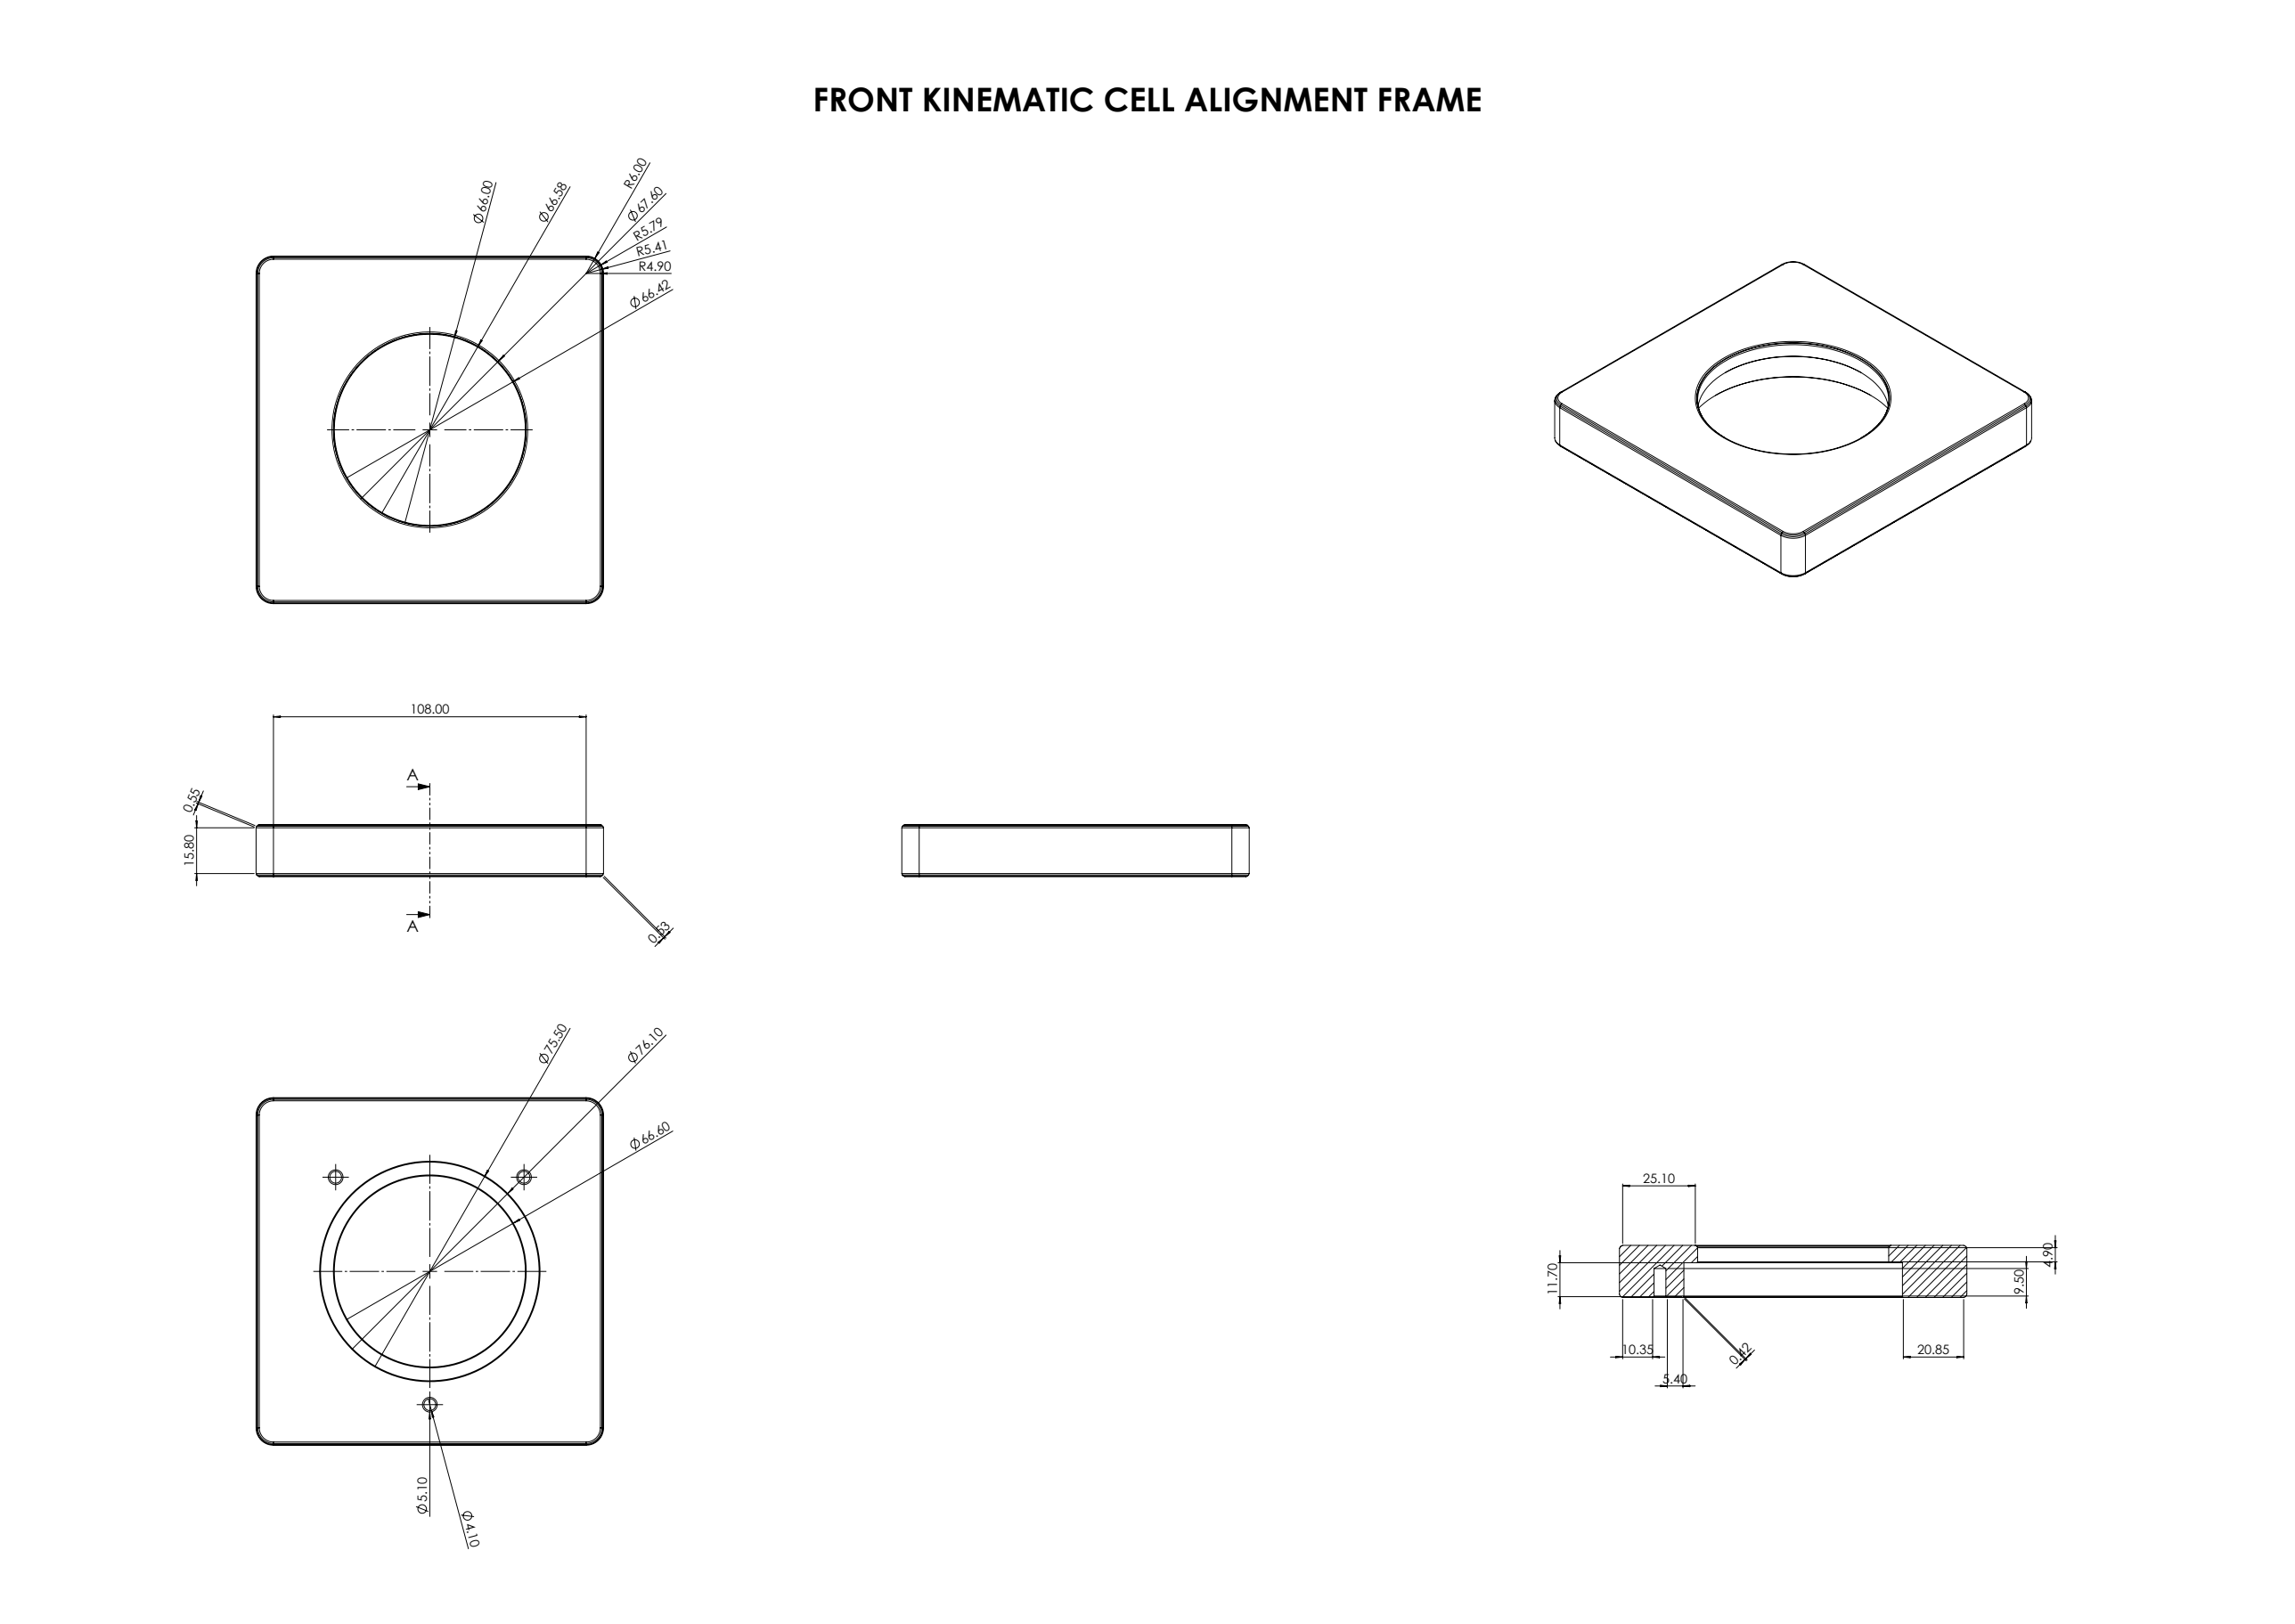
ISO-10303-21;
HEADER;
/* Generated by software containing ST-Developer
 * from STEP Tools, Inc. (www.steptools.com) 
 */

FILE_DESCRIPTION(
/* description */ (''),
/* implementation_level */ '2;1');

FILE_NAME(
/* name */ '03_Front_Kinematic_Cell_Alignment_Frame.step',
/* time_stamp */ '2026-10-19T22:59:19-07:00',
/* author */ (''),
/* organization */ (''),
/* preprocessor_version */ 'ST-DEVELOPER v20.2',
/* originating_system */ 'Autodesk Translation Framework v15.15.0.0',
/* authorisation */ '');

FILE_SCHEMA (('AUTOMOTIVE_DESIGN { 1 0 10303 214 3 1 1 }'));
ENDSEC;

DATA;
#10=MECHANICAL_DESIGN_GEOMETRIC_PRESENTATION_REPRESENTATION('',(#913),#53650);
#881=SHAPE_REPRESENTATION_RELATIONSHIP('SRR','None',#53726,#897);
#897=ADVANCED_BREP_SHAPE_REPRESENTATION('',(#929),#53636);
#913=STYLED_ITEM('',(#53937),#929);
#929=MANIFOLD_SOLID_BREP('Front Cell Alignment Frame',#23305);
#978=CYLINDRICAL_SURFACE('',#23898,0.6);
#979=CYLINDRICAL_SURFACE('',#23901,0.6);
#980=CYLINDRICAL_SURFACE('',#23929,3.775);
#981=CYLINDRICAL_SURFACE('',#23953,3.3);
#982=CYLINDRICAL_SURFACE('',#23963,0.205);
#983=CYLINDRICAL_SURFACE('',#23968,0.205);
#984=CYLINDRICAL_SURFACE('',#23973,0.205);
#985=CYLINDRICAL_SURFACE('',#23980,0.6);
#986=CYLINDRICAL_SURFACE('',#23982,0.6);
#1320=FACE_BOUND('',#3813,.T.);
#1321=FACE_BOUND('',#3814,.T.);
#1322=FACE_BOUND('',#3815,.T.);
#1323=FACE_BOUND('',#3816,.T.);
#1324=FACE_BOUND('',#3857,.T.);
#1325=FACE_BOUND('',#3861,.T.);
#1518=PLANE('',#23860);
#1519=PLANE('',#23864);
#1520=PLANE('',#23868);
#1521=PLANE('',#23872);
#1522=PLANE('',#23873);
#1523=PLANE('',#23876);
#1524=PLANE('',#23879);
#1525=PLANE('',#23884);
#1526=PLANE('',#23888);
#1527=PLANE('',#23891);
#1528=PLANE('',#23894);
#1529=PLANE('',#23900);
#1530=PLANE('',#23903);
#1531=PLANE('',#23905);
#1532=PLANE('',#23908);
#1533=PLANE('',#23911);
#1534=PLANE('',#23915);
#1535=PLANE('',#23919);
#1536=PLANE('',#23920);
#1537=PLANE('',#23923);
#1538=PLANE('',#23933);
#1539=PLANE('',#23936);
#1540=PLANE('',#23940);
#1541=PLANE('',#23944);
#1542=PLANE('',#23945);
#1543=PLANE('',#23947);
#1544=PLANE('',#23948);
#1545=PLANE('',#23955);
#1546=PLANE('',#23977);
#1547=PLANE('',#23979);
#1548=PLANE('',#23981);
#2429=FACE_OUTER_BOUND('',#3800,.T.);
#2430=FACE_OUTER_BOUND('',#3801,.T.);
#2431=FACE_OUTER_BOUND('',#3802,.T.);
#2432=FACE_OUTER_BOUND('',#3803,.T.);
#2433=FACE_OUTER_BOUND('',#3804,.T.);
#2434=FACE_OUTER_BOUND('',#3805,.T.);
#2435=FACE_OUTER_BOUND('',#3806,.T.);
#2436=FACE_OUTER_BOUND('',#3807,.T.);
#2437=FACE_OUTER_BOUND('',#3808,.T.);
#2438=FACE_OUTER_BOUND('',#3809,.T.);
#2439=FACE_OUTER_BOUND('',#3810,.T.);
#2440=FACE_OUTER_BOUND('',#3811,.T.);
#2441=FACE_OUTER_BOUND('',#3812,.T.);
#2442=FACE_OUTER_BOUND('',#3817,.T.);
#2443=FACE_OUTER_BOUND('',#3818,.T.);
#2444=FACE_OUTER_BOUND('',#3819,.T.);
#2445=FACE_OUTER_BOUND('',#3820,.T.);
#2446=FACE_OUTER_BOUND('',#3821,.T.);
#2447=FACE_OUTER_BOUND('',#3822,.T.);
#2448=FACE_OUTER_BOUND('',#3823,.T.);
#2449=FACE_OUTER_BOUND('',#3824,.T.);
#2450=FACE_OUTER_BOUND('',#3825,.T.);
#2451=FACE_OUTER_BOUND('',#3826,.T.);
#2452=FACE_OUTER_BOUND('',#3827,.T.);
#2453=FACE_OUTER_BOUND('',#3828,.T.);
#2454=FACE_OUTER_BOUND('',#3829,.T.);
#2455=FACE_OUTER_BOUND('',#3830,.T.);
#2456=FACE_OUTER_BOUND('',#3831,.T.);
#2457=FACE_OUTER_BOUND('',#3832,.T.);
#2458=FACE_OUTER_BOUND('',#3833,.T.);
#2459=FACE_OUTER_BOUND('',#3834,.T.);
#2460=FACE_OUTER_BOUND('',#3835,.T.);
#2461=FACE_OUTER_BOUND('',#3836,.T.);
#2462=FACE_OUTER_BOUND('',#3837,.T.);
#2463=FACE_OUTER_BOUND('',#3838,.T.);
#2464=FACE_OUTER_BOUND('',#3839,.T.);
#2465=FACE_OUTER_BOUND('',#3840,.T.);
#2466=FACE_OUTER_BOUND('',#3841,.T.);
#2467=FACE_OUTER_BOUND('',#3842,.T.);
#2468=FACE_OUTER_BOUND('',#3843,.T.);
#2469=FACE_OUTER_BOUND('',#3844,.T.);
#2470=FACE_OUTER_BOUND('',#3845,.T.);
#2471=FACE_OUTER_BOUND('',#3846,.T.);
#2472=FACE_OUTER_BOUND('',#3847,.T.);
#2473=FACE_OUTER_BOUND('',#3848,.T.);
#2474=FACE_OUTER_BOUND('',#3849,.T.);
#2475=FACE_OUTER_BOUND('',#3850,.T.);
#2476=FACE_OUTER_BOUND('',#3851,.T.);
#2477=FACE_OUTER_BOUND('',#3852,.T.);
#2478=FACE_OUTER_BOUND('',#3853,.T.);
#2479=FACE_OUTER_BOUND('',#3854,.T.);
#2480=FACE_OUTER_BOUND('',#3855,.T.);
#2481=FACE_OUTER_BOUND('',#3856,.T.);
#2482=FACE_OUTER_BOUND('',#3858,.T.);
#2483=FACE_OUTER_BOUND('',#3859,.T.);
#2484=FACE_OUTER_BOUND('',#3860,.T.);
#2485=FACE_OUTER_BOUND('',#3862,.T.);
#2486=FACE_OUTER_BOUND('',#3863,.T.);
#2487=FACE_OUTER_BOUND('',#3864,.T.);
#2488=FACE_OUTER_BOUND('',#3865,.T.);
#2489=FACE_OUTER_BOUND('',#3866,.T.);
#2490=FACE_OUTER_BOUND('',#3867,.T.);
#2491=FACE_OUTER_BOUND('',#3868,.T.);
#2492=FACE_OUTER_BOUND('',#3869,.T.);
#2493=FACE_OUTER_BOUND('',#3870,.T.);
#2494=FACE_OUTER_BOUND('',#3871,.T.);
#2495=FACE_OUTER_BOUND('',#3872,.T.);
#2496=FACE_OUTER_BOUND('',#3873,.T.);
#2497=FACE_OUTER_BOUND('',#3874,.T.);
#2498=FACE_OUTER_BOUND('',#3875,.T.);
#2499=FACE_OUTER_BOUND('',#3876,.T.);
#2500=FACE_OUTER_BOUND('',#3877,.T.);
#2501=FACE_OUTER_BOUND('',#3878,.T.);
#2502=FACE_OUTER_BOUND('',#3879,.T.);
#2503=FACE_OUTER_BOUND('',#3880,.T.);
#3800=EDGE_LOOP('',(#15901,#15902,#15903,#15904));
#3801=EDGE_LOOP('',(#15905,#15906,#15907,#15908));
#3802=EDGE_LOOP('',(#15909,#15910,#15911,#15912));
#3803=EDGE_LOOP('',(#15913,#15914,#15915,#15916));
#3804=EDGE_LOOP('',(#15917,#15918,#15919,#15920));
#3805=EDGE_LOOP('',(#15921,#15922,#15923,#15924));
#3806=EDGE_LOOP('',(#15925,#15926,#15927,#15928));
#3807=EDGE_LOOP('',(#15929,#15930,#15931,#15932));
#3808=EDGE_LOOP('',(#15933,#15934,#15935,#15936));
#3809=EDGE_LOOP('',(#15937,#15938,#15939,#15940));
#3810=EDGE_LOOP('',(#15941,#15942,#15943,#15944));
#3811=EDGE_LOOP('',(#15945,#15946,#15947,#15948));
#3812=EDGE_LOOP('',(#15949,#15950,#15951,#15952,#15953,#15954,#15955,#15956));
#3813=EDGE_LOOP('',(#15957));
#3814=EDGE_LOOP('',(#15958));
#3815=EDGE_LOOP('',(#15959));
#3816=EDGE_LOOP('',(#15960));
#3817=EDGE_LOOP('',(#15961,#15962,#15963,#15964));
#3818=EDGE_LOOP('',(#15965,#15966,#15967,#15968));
#3819=EDGE_LOOP('',(#15969,#15970,#15971,#15972));
#3820=EDGE_LOOP('',(#15973,#15974,#15975,#15976));
#3821=EDGE_LOOP('',(#15977,#15978,#15979,#15980));
#3822=EDGE_LOOP('',(#15981,#15982,#15983,#15984));
#3823=EDGE_LOOP('',(#15985,#15986,#15987,#15988));
#3824=EDGE_LOOP('',(#15989,#15990,#15991,#15992));
#3825=EDGE_LOOP('',(#15993,#15994,#15995,#15996));
#3826=EDGE_LOOP('',(#15997,#15998,#15999,#16000));
#3827=EDGE_LOOP('',(#16001,#16002,#16003,#16004));
#3828=EDGE_LOOP('',(#16005,#16006,#16007,#16008));
#3829=EDGE_LOOP('',(#16009,#16010,#16011,#16012));
#3830=EDGE_LOOP('',(#16013,#16014,#16015,#16016));
#3831=EDGE_LOOP('',(#16017,#16018,#16019,#16020));
#3832=EDGE_LOOP('',(#16021,#16022,#16023,#16024));
#3833=EDGE_LOOP('',(#16025,#16026,#16027,#16028));
#3834=EDGE_LOOP('',(#16029,#16030,#16031,#16032));
#3835=EDGE_LOOP('',(#16033,#16034,#16035,#16036));
#3836=EDGE_LOOP('',(#16037,#16038,#16039,#16040));
#3837=EDGE_LOOP('',(#16041,#16042,#16043,#16044));
#3838=EDGE_LOOP('',(#16045,#16046,#16047,#16048));
#3839=EDGE_LOOP('',(#16049,#16050,#16051,#16052));
#3840=EDGE_LOOP('',(#16053,#16054,#16055,#16056));
#3841=EDGE_LOOP('',(#16057,#16058,#16059,#16060));
#3842=EDGE_LOOP('',(#16061,#16062,#16063,#16064));
#3843=EDGE_LOOP('',(#16065,#16066,#16067,#16068,#16069));
#3844=EDGE_LOOP('',(#16070,#16071,#16072,#16073,#16074));
#3845=EDGE_LOOP('',(#16075,#16076,#16077,#16078));
#3846=EDGE_LOOP('',(#16079,#16080,#16081,#16082));
#3847=EDGE_LOOP('',(#16083,#16084,#16085,#16086));
#3848=EDGE_LOOP('',(#16087,#16088,#16089,#16090));
#3849=EDGE_LOOP('',(#16091,#16092,#16093,#16094));
#3850=EDGE_LOOP('',(#16095,#16096,#16097,#16098));
#3851=EDGE_LOOP('',(#16099,#16100,#16101,#16102));
#3852=EDGE_LOOP('',(#16103,#16104,#16105,#16106));
#3853=EDGE_LOOP('',(#16107,#16108,#16109,#16110));
#3854=EDGE_LOOP('',(#16111,#16112,#16113,#16114));
#3855=EDGE_LOOP('',(#16115,#16116,#16117,#16118));
#3856=EDGE_LOOP('',(#16119,#16120,#16121,#16122,#16123,#16124,#16125,#16126));
#3857=EDGE_LOOP('',(#16127));
#3858=EDGE_LOOP('',(#16128,#16129,#16130,#16131));
#3859=EDGE_LOOP('',(#16132,#16133,#16134,#16135));
#3860=EDGE_LOOP('',(#16136));
#3861=EDGE_LOOP('',(#16137));
#3862=EDGE_LOOP('',(#16138,#16139,#16140,#16141));
#3863=EDGE_LOOP('',(#16142,#16143,#16144,#16145));
#3864=EDGE_LOOP('',(#16146,#16147,#16148,#16149));
#3865=EDGE_LOOP('',(#16150,#16151,#16152));
#3866=EDGE_LOOP('',(#16153,#16154,#16155,#16156));
#3867=EDGE_LOOP('',(#16157,#16158,#16159,#16160));
#3868=EDGE_LOOP('',(#16161,#16162,#16163));
#3869=EDGE_LOOP('',(#16164,#16165,#16166,#16167));
#3870=EDGE_LOOP('',(#16168,#16169,#16170,#16171));
#3871=EDGE_LOOP('',(#16172,#16173,#16174));
#3872=EDGE_LOOP('',(#16175,#16176,#16177,#16178));
#3873=EDGE_LOOP('',(#16179,#16180,#16181,#16182));
#3874=EDGE_LOOP('',(#16183,#16184,#16185,#16186));
#3875=EDGE_LOOP('',(#16187,#16188,#16189,#16190));
#3876=EDGE_LOOP('',(#16191,#16192,#16193,#16194));
#3877=EDGE_LOOP('',(#16195,#16196,#16197,#16198));
#3878=EDGE_LOOP('',(#16199,#16200,#16201,#16202));
#3879=EDGE_LOOP('',(#16203,#16204,#16205,#16206));
#3880=EDGE_LOOP('',(#16207,#16208,#16209,#16210));
#5227=CIRCLE('',#23858,0.541213203435597);
#5228=CIRCLE('',#23859,0.49);
#5229=CIRCLE('',#23862,0.541213203435597);
#5230=CIRCLE('',#23863,0.49);
#5231=CIRCLE('',#23866,0.541213203435597);
#5232=CIRCLE('',#23867,0.49);
#5233=CIRCLE('',#23870,0.541213203435596);
#5234=CIRCLE('',#23871,0.489999999999999);
#5235=CIRCLE('',#23875,0.578786796564404);
#5236=CIRCLE('',#23878,0.578786796564403);
#5237=CIRCLE('',#23880,3.805);
#5238=CIRCLE('',#23881,0.255);
#5239=CIRCLE('',#23882,0.255);
#5240=CIRCLE('',#23883,0.255);
#5241=CIRCLE('',#23886,0.578786796564403);
#5242=CIRCLE('',#23887,0.6);
#5243=CIRCLE('',#23890,0.6);
#5244=CIRCLE('',#23893,0.6);
#5245=CIRCLE('',#23896,0.578786796564403);
#5246=CIRCLE('',#23897,0.6);
#5247=CIRCLE('',#23899,0.6);
#5248=CIRCLE('',#23902,0.6);
#5249=CIRCLE('',#23907,0.578786796564403);
#5250=CIRCLE('',#23910,0.578786796564404);
#5251=CIRCLE('',#23913,0.578786796564404);
#5252=CIRCLE('',#23914,0.6);
#5253=CIRCLE('',#23917,0.578786796564404);
#5254=CIRCLE('',#23918,0.6);
#5255=CIRCLE('',#23922,0.541213203435596);
#5256=CIRCLE('',#23925,0.541213203435597);
#5257=CIRCLE('',#23927,3.775);
#5258=CIRCLE('',#23928,3.775);
#5259=CIRCLE('',#23930,3.775);
#5260=CIRCLE('',#23932,0.49);
#5261=CIRCLE('',#23935,0.489999999999998);
#5262=CIRCLE('',#23938,0.541213203435597);
#5263=CIRCLE('',#23939,0.49);
#5264=CIRCLE('',#23942,0.541213203435597);
#5265=CIRCLE('',#23943,0.49);
#5266=CIRCLE('',#23949,3.38);
#5267=CIRCLE('',#23951,3.3);
#5268=CIRCLE('',#23952,3.33);
#5269=CIRCLE('',#23954,3.3);
#5270=CIRCLE('',#23957,3.3287867965644);
#5271=CIRCLE('',#23959,3.3212132034356);
#5272=CIRCLE('',#23962,0.205);
#5273=CIRCLE('',#23964,0.205);
#5274=CIRCLE('',#23967,0.205);
#5275=CIRCLE('',#23969,0.205);
#5276=CIRCLE('',#23972,0.205);
#5277=CIRCLE('',#23974,0.205);
#6105=LINE('',#32675,#7950);
#6106=LINE('',#32679,#7951);
#6107=LINE('',#32684,#7952);
#6108=LINE('',#32685,#7953);
#6109=LINE('',#32686,#7954);
#6110=LINE('',#32690,#7955);
#6111=LINE('',#32696,#7956);
#6112=LINE('',#32697,#7957);
#6113=LINE('',#32698,#7958);
#6114=LINE('',#32702,#7959);
#6115=LINE('',#32708,#7960);
#6116=LINE('',#32709,#7961);
#6117=LINE('',#32710,#7962);
#6118=LINE('',#32714,#7963);
#6119=LINE('',#32718,#7964);
#6120=LINE('',#32719,#7965);
#6121=LINE('',#32722,#7966);
#6122=LINE('',#32724,#7967);
#6123=LINE('',#32725,#7968);
#6124=LINE('',#32728,#7969);
#6125=LINE('',#32732,#7970);
#6126=LINE('',#32733,#7971);
#6127=LINE('',#32736,#7972);
#6128=LINE('',#32750,#7973);
#6129=LINE('',#32752,#7974);
#6130=LINE('',#32754,#7975);
#6131=LINE('',#32755,#7976);
#6132=LINE('',#32759,#7977);
#6133=LINE('',#32764,#7978);
#6134=LINE('',#32765,#7979);
#6135=LINE('',#32766,#7980);
#6136=LINE('',#32769,#7981);
#6137=LINE('',#32773,#7982);
#6138=LINE('',#32774,#7983);
#6139=LINE('',#32777,#7984);
#6140=LINE('',#32781,#7985);
#6141=LINE('',#32782,#7986);
#6142=LINE('',#32788,#7987);
#6143=LINE('',#32791,#7988);
#6144=LINE('',#32794,#7989);
#6145=LINE('',#32795,#7990);
#6146=LINE('',#32798,#7991);
#6147=LINE('',#32802,#7992);
#6148=LINE('',#32803,#7993);
#6149=LINE('',#32805,#7994);
#6150=LINE('',#32807,#7995);
#6151=LINE('',#32810,#7996);
#6152=LINE('',#32813,#7997);
#6153=LINE('',#32816,#7998);
#6154=LINE('',#32817,#7999);
#6155=LINE('',#32820,#8000);
#6156=LINE('',#32824,#8001);
#6157=LINE('',#32825,#8002);
#6158=LINE('',#32829,#8003);
#6159=LINE('',#32835,#8004);
#6160=LINE('',#32836,#8005);
#6161=LINE('',#32837,#8006);
#6162=LINE('',#32841,#8007);
#6163=LINE('',#32845,#8008);
#6164=LINE('',#32846,#8009);
#6165=LINE('',#32849,#8010);
#6166=LINE('',#32851,#8011);
#6167=LINE('',#32852,#8012);
#6168=LINE('',#32855,#8013);
#6169=LINE('',#32859,#8014);
#6170=LINE('',#32860,#8015);
#6171=LINE('',#32863,#8016);
#6172=LINE('',#32867,#8017);
#6173=LINE('',#32874,#8018);
#6174=LINE('',#32877,#8019);
#6175=LINE('',#32879,#8020);
#6176=LINE('',#32883,#8021);
#6177=LINE('',#32884,#8022);
#6178=LINE('',#32887,#8023);
#6179=LINE('',#32891,#8024);
#6180=LINE('',#32892,#8025);
#6181=LINE('',#32896,#8026);
#6182=LINE('',#32902,#8027);
#6183=LINE('',#32903,#8028);
#6184=LINE('',#32904,#8029);
#6185=LINE('',#32908,#8030);
#6186=LINE('',#32912,#8031);
#6187=LINE('',#32913,#8032);
#6188=LINE('',#32915,#8033);
#6189=LINE('',#32916,#8034);
#6190=LINE('',#32918,#8035);
#6191=LINE('',#32927,#8036);
#6192=LINE('',#32932,#8037);
#6193=LINE('',#32937,#8038);
#6194=LINE('',#32940,#8039);
#6195=LINE('',#32943,#8040);
#6196=LINE('',#32947,#8041);
#6197=LINE('',#32951,#8042);
#6198=LINE('',#32954,#8043);
#6199=LINE('',#32958,#8044);
#6200=LINE('',#32962,#8045);
#6201=LINE('',#32965,#8046);
#6202=LINE('',#32969,#8047);
#6203=LINE('',#32973,#8048);
#6204=LINE('',#32976,#8049);
#6205=LINE('',#32979,#8050);
#6206=LINE('',#32982,#8051);
#6207=LINE('',#32983,#8052);
#6208=LINE('',#32985,#8053);
#7950=VECTOR('',#26631,1.);
#7951=VECTOR('',#26634,1.);
#7952=VECTOR('',#26639,1.);
#7953=VECTOR('',#26640,1.);
#7954=VECTOR('',#26641,1.);
#7955=VECTOR('',#26644,1.);
#7956=VECTOR('',#26651,1.);
#7957=VECTOR('',#26652,1.);
#7958=VECTOR('',#26653,1.);
#7959=VECTOR('',#26656,1.);
#7960=VECTOR('',#26663,1.);
#7961=VECTOR('',#26664,1.);
#7962=VECTOR('',#26665,1.);
#7963=VECTOR('',#26668,1.);
#7964=VECTOR('',#26675,1.);
#7965=VECTOR('',#26676,1.);
#7966=VECTOR('',#26679,1.);
#7967=VECTOR('',#26680,1.);
#7968=VECTOR('',#26681,1.);
#7969=VECTOR('',#26684,1.);
#7970=VECTOR('',#26689,1.);
#7971=VECTOR('',#26690,1.);
#7972=VECTOR('',#26693,1.);
#7973=VECTOR('',#26708,1.);
#7974=VECTOR('',#26709,1.);
#7975=VECTOR('',#26710,1.);
#7976=VECTOR('',#26711,1.);
#7977=VECTOR('',#26714,1.);
#7978=VECTOR('',#26721,1.);
#7979=VECTOR('',#26722,1.);
#7980=VECTOR('',#26723,1.);
#7981=VECTOR('',#26726,1.);
#7982=VECTOR('',#26731,1.);
#7983=VECTOR('',#26732,1.);
#7984=VECTOR('',#26735,1.);
#7985=VECTOR('',#26740,1.);
#7986=VECTOR('',#26741,1.);
#7987=VECTOR('',#26750,1.);
#7988=VECTOR('',#26753,1.);
#7989=VECTOR('',#26756,1.);
#7990=VECTOR('',#26757,1.);
#7991=VECTOR('',#26760,1.);
#7992=VECTOR('',#26765,1.);
#7993=VECTOR('',#26766,1.);
#7994=VECTOR('',#26769,1.);
#7995=VECTOR('',#26772,1.);
#7996=VECTOR('',#26775,1.);
#7997=VECTOR('',#26778,1.);
#7998=VECTOR('',#26781,1.);
#7999=VECTOR('',#26782,1.);
#8000=VECTOR('',#26785,1.);
#8001=VECTOR('',#26790,1.);
#8002=VECTOR('',#26791,1.);
#8003=VECTOR('',#26794,1.);
#8004=VECTOR('',#26801,1.);
#8005=VECTOR('',#26802,1.);
#8006=VECTOR('',#26803,1.);
#8007=VECTOR('',#26806,1.);
#8008=VECTOR('',#26813,1.);
#8009=VECTOR('',#26814,1.);
#8010=VECTOR('',#26817,1.);
#8011=VECTOR('',#26818,1.);
#8012=VECTOR('',#26819,1.);
#8013=VECTOR('',#26822,1.);
#8014=VECTOR('',#26827,1.);
#8015=VECTOR('',#26828,1.);
#8016=VECTOR('',#26831,1.);
#8017=VECTOR('',#26836,3.79);
#8018=VECTOR('',#26845,3.775);
#8019=VECTOR('',#26848,1.);
#8020=VECTOR('',#26849,1.);
#8021=VECTOR('',#26854,1.);
#8022=VECTOR('',#26855,1.);
#8023=VECTOR('',#26858,1.);
#8024=VECTOR('',#26863,1.);
#8025=VECTOR('',#26864,1.);
#8026=VECTOR('',#26867,1.);
#8027=VECTOR('',#26874,1.);
#8028=VECTOR('',#26875,1.);
#8029=VECTOR('',#26876,1.);
#8030=VECTOR('',#26879,1.);
#8031=VECTOR('',#26886,1.);
#8032=VECTOR('',#26887,1.);
#8033=VECTOR('',#26890,1.);
#8034=VECTOR('',#26891,1.);
#8035=VECTOR('',#26894,1.);
#8036=VECTOR('',#26905,3.315);
#8037=VECTOR('',#26912,3.3);
#8038=VECTOR('',#26919,3.3543933982822);
#8039=VECTOR('',#26922,3.325);
#8040=VECTOR('',#26927,3.3106066017178);
#8041=VECTOR('',#26930,0.1025);
#8042=VECTOR('',#26935,0.205);
#8043=VECTOR('',#26940,0.255);
#8044=VECTOR('',#26943,0.1025);
#8045=VECTOR('',#26948,0.205);
#8046=VECTOR('',#26953,0.255);
#8047=VECTOR('',#26956,0.1025);
#8048=VECTOR('',#26961,0.205);
#8049=VECTOR('',#26966,0.255);
#8050=VECTOR('',#26971,1.);
#8051=VECTOR('',#26976,1.);
#8052=VECTOR('',#26977,1.);
#8053=VECTOR('',#26980,1.);
#9785=VERTEX_POINT('',#32673);
#9786=VERTEX_POINT('',#32674);
#9787=VERTEX_POINT('',#32676);
#9788=VERTEX_POINT('',#32678);
#9789=VERTEX_POINT('',#32682);
#9790=VERTEX_POINT('',#32683);
#9791=VERTEX_POINT('',#32688);
#9792=VERTEX_POINT('',#32689);
#9793=VERTEX_POINT('',#32694);
#9794=VERTEX_POINT('',#32695);
#9795=VERTEX_POINT('',#32700);
#9796=VERTEX_POINT('',#32701);
#9797=VERTEX_POINT('',#32706);
#9798=VERTEX_POINT('',#32707);
#9799=VERTEX_POINT('',#32712);
#9800=VERTEX_POINT('',#32713);
#9801=VERTEX_POINT('',#32721);
#9802=VERTEX_POINT('',#32723);
#9803=VERTEX_POINT('',#32727);
#9804=VERTEX_POINT('',#32731);
#9805=VERTEX_POINT('',#32735);
#9806=VERTEX_POINT('',#32739);
#9807=VERTEX_POINT('',#32741);
#9808=VERTEX_POINT('',#32743);
#9809=VERTEX_POINT('',#32745);
#9810=VERTEX_POINT('',#32748);
#9811=VERTEX_POINT('',#32749);
#9812=VERTEX_POINT('',#32751);
#9813=VERTEX_POINT('',#32753);
#9814=VERTEX_POINT('',#32757);
#9815=VERTEX_POINT('',#32758);
#9816=VERTEX_POINT('',#32763);
#9817=VERTEX_POINT('',#32768);
#9818=VERTEX_POINT('',#32772);
#9819=VERTEX_POINT('',#32776);
#9820=VERTEX_POINT('',#32780);
#9821=VERTEX_POINT('',#32787);
#9822=VERTEX_POINT('',#32789);
#9823=VERTEX_POINT('',#32793);
#9824=VERTEX_POINT('',#32797);
#9825=VERTEX_POINT('',#32801);
#9826=VERTEX_POINT('',#32809);
#9827=VERTEX_POINT('',#32811);
#9828=VERTEX_POINT('',#32815);
#9829=VERTEX_POINT('',#32819);
#9830=VERTEX_POINT('',#32823);
#9831=VERTEX_POINT('',#32827);
#9832=VERTEX_POINT('',#32828);
#9833=VERTEX_POINT('',#32833);
#9834=VERTEX_POINT('',#32834);
#9835=VERTEX_POINT('',#32839);
#9836=VERTEX_POINT('',#32840);
#9837=VERTEX_POINT('',#32848);
#9838=VERTEX_POINT('',#32850);
#9839=VERTEX_POINT('',#32854);
#9840=VERTEX_POINT('',#32858);
#9841=VERTEX_POINT('',#32862);
#9842=VERTEX_POINT('',#32866);
#9843=VERTEX_POINT('',#32868);
#9844=VERTEX_POINT('',#32872);
#9845=VERTEX_POINT('',#32876);
#9846=VERTEX_POINT('',#32878);
#9847=VERTEX_POINT('',#32882);
#9848=VERTEX_POINT('',#32886);
#9849=VERTEX_POINT('',#32890);
#9850=VERTEX_POINT('',#32894);
#9851=VERTEX_POINT('',#32895);
#9852=VERTEX_POINT('',#32900);
#9853=VERTEX_POINT('',#32901);
#9854=VERTEX_POINT('',#32906);
#9855=VERTEX_POINT('',#32907);
#9856=VERTEX_POINT('',#32921);
#9857=VERTEX_POINT('',#32924);
#9858=VERTEX_POINT('',#32926);
#9859=VERTEX_POINT('',#32930);
#9860=VERTEX_POINT('',#32935);
#9861=VERTEX_POINT('',#32939);
#9862=VERTEX_POINT('',#32945);
#9863=VERTEX_POINT('',#32946);
#9864=VERTEX_POINT('',#32950);
#9865=VERTEX_POINT('',#32956);
#9866=VERTEX_POINT('',#32957);
#9867=VERTEX_POINT('',#32961);
#9868=VERTEX_POINT('',#32967);
#9869=VERTEX_POINT('',#32968);
#9870=VERTEX_POINT('',#32972);
#12128=EDGE_CURVE('',#9785,#9786,#6105,.T.);
#12129=EDGE_CURVE('',#9786,#9787,#5227,.T.);
#12130=EDGE_CURVE('',#9787,#9788,#6106,.T.);
#12131=EDGE_CURVE('',#9788,#9785,#5228,.T.);
#12132=EDGE_CURVE('',#9789,#9790,#6107,.T.);
#12133=EDGE_CURVE('',#9790,#9786,#6108,.T.);
#12134=EDGE_CURVE('',#9785,#9789,#6109,.T.);
#12135=EDGE_CURVE('',#9791,#9792,#6110,.T.);
#12136=EDGE_CURVE('',#9792,#9790,#5229,.T.);
#12137=EDGE_CURVE('',#9789,#9791,#5230,.T.);
#12138=EDGE_CURVE('',#9793,#9794,#6111,.T.);
#12139=EDGE_CURVE('',#9794,#9792,#6112,.T.);
#12140=EDGE_CURVE('',#9791,#9793,#6113,.T.);
#12141=EDGE_CURVE('',#9795,#9796,#6114,.T.);
#12142=EDGE_CURVE('',#9796,#9794,#5231,.T.);
#12143=EDGE_CURVE('',#9793,#9795,#5232,.T.);
#12144=EDGE_CURVE('',#9797,#9798,#6115,.T.);
#12145=EDGE_CURVE('',#9798,#9796,#6116,.T.);
#12146=EDGE_CURVE('',#9795,#9797,#6117,.T.);
#12147=EDGE_CURVE('',#9799,#9800,#6118,.T.);
#12148=EDGE_CURVE('',#9800,#9798,#5233,.T.);
#12149=EDGE_CURVE('',#9797,#9799,#5234,.T.);
#12150=EDGE_CURVE('',#9787,#9800,#6119,.T.);
#12151=EDGE_CURVE('',#9799,#9788,#6120,.T.);
#12152=EDGE_CURVE('',#9798,#9801,#6121,.T.);
#12153=EDGE_CURVE('',#9802,#9801,#6122,.T.);
#12154=EDGE_CURVE('',#9796,#9802,#6123,.T.);
#12155=EDGE_CURVE('',#9800,#9803,#6124,.T.);
#12156=EDGE_CURVE('',#9801,#9803,#5235,.T.);
#12157=EDGE_CURVE('',#9804,#9787,#6125,.T.);
#12158=EDGE_CURVE('',#9803,#9804,#6126,.T.);
#12159=EDGE_CURVE('',#9786,#9805,#6127,.T.);
#12160=EDGE_CURVE('',#9804,#9805,#5236,.T.);
#12161=EDGE_CURVE('',#9806,#9806,#5237,.T.);
#12162=EDGE_CURVE('',#9807,#9807,#5238,.T.);
#12163=EDGE_CURVE('',#9808,#9808,#5239,.T.);
#12164=EDGE_CURVE('',#9809,#9809,#5240,.T.);
#12165=EDGE_CURVE('',#9810,#9811,#6128,.T.);
#12166=EDGE_CURVE('',#9811,#9812,#6129,.T.);
#12167=EDGE_CURVE('',#9812,#9813,#6130,.T.);
#12168=EDGE_CURVE('',#9813,#9810,#6131,.T.);
#12169=EDGE_CURVE('',#9814,#9815,#6132,.T.);
#12170=EDGE_CURVE('',#9815,#9811,#5241,.T.);
#12171=EDGE_CURVE('',#9810,#9814,#5242,.T.);
#12172=EDGE_CURVE('',#9816,#9805,#6133,.T.);
#12173=EDGE_CURVE('',#9805,#9815,#6134,.T.);
#12174=EDGE_CURVE('',#9814,#9816,#6135,.T.);
#12175=EDGE_CURVE('',#9817,#9804,#6136,.T.);
#12176=EDGE_CURVE('',#9816,#9817,#5243,.T.);
#12177=EDGE_CURVE('',#9818,#9803,#6137,.T.);
#12178=EDGE_CURVE('',#9817,#9818,#6138,.T.);
#12179=EDGE_CURVE('',#9819,#9801,#6139,.T.);
#12180=EDGE_CURVE('',#9818,#9819,#5244,.T.);
#12181=EDGE_CURVE('',#9820,#9802,#6140,.T.);
#12182=EDGE_CURVE('',#9819,#9820,#6141,.T.);
#12183=EDGE_CURVE('',#9812,#9802,#5245,.T.);
#12184=EDGE_CURVE('',#9820,#9813,#5246,.T.);
#12185=EDGE_CURVE('',#9816,#9821,#6142,.T.);
#12186=EDGE_CURVE('',#9822,#9821,#5247,.T.);
#12187=EDGE_CURVE('',#9822,#9817,#6143,.T.);
#12188=EDGE_CURVE('',#9823,#9814,#6144,.T.);
#12189=EDGE_CURVE('',#9821,#9823,#6145,.T.);
#12190=EDGE_CURVE('',#9810,#9824,#6146,.T.);
#12191=EDGE_CURVE('',#9823,#9824,#5248,.T.);
#12192=EDGE_CURVE('',#9825,#9813,#6147,.T.);
#12193=EDGE_CURVE('',#9824,#9825,#6148,.T.);
#12194=EDGE_CURVE('',#9794,#9812,#6149,.T.);
#12195=EDGE_CURVE('',#9792,#9811,#6150,.T.);
#12196=EDGE_CURVE('',#9821,#9826,#6151,.T.);
#12197=EDGE_CURVE('',#9826,#9827,#5249,.T.);
#12198=EDGE_CURVE('',#9827,#9822,#6152,.T.);
#12199=EDGE_CURVE('',#9823,#9828,#6153,.T.);
#12200=EDGE_CURVE('',#9828,#9826,#6154,.T.);
#12201=EDGE_CURVE('',#9824,#9829,#6155,.T.);
#12202=EDGE_CURVE('',#9829,#9828,#5250,.T.);
#12203=EDGE_CURVE('',#9825,#9830,#6156,.T.);
#12204=EDGE_CURVE('',#9830,#9829,#6157,.T.);
#12205=EDGE_CURVE('',#9831,#9832,#6158,.T.);
#12206=EDGE_CURVE('',#9832,#9830,#5251,.T.);
#12207=EDGE_CURVE('',#9825,#9831,#5252,.T.);
#12208=EDGE_CURVE('',#9833,#9834,#6159,.T.);
#12209=EDGE_CURVE('',#9834,#9832,#6160,.T.);
#12210=EDGE_CURVE('',#9831,#9833,#6161,.T.);
#12211=EDGE_CURVE('',#9835,#9836,#6162,.T.);
#12212=EDGE_CURVE('',#9836,#9834,#5253,.T.);
#12213=EDGE_CURVE('',#9833,#9835,#5254,.T.);
#12214=EDGE_CURVE('',#9827,#9836,#6163,.T.);
#12215=EDGE_CURVE('',#9835,#9822,#6164,.T.);
#12216=EDGE_CURVE('',#9837,#9834,#6165,.T.);
#12217=EDGE_CURVE('',#9838,#9837,#6166,.T.);
#12218=EDGE_CURVE('',#9838,#9832,#6167,.T.);
#12219=EDGE_CURVE('',#9839,#9836,#6168,.T.);
#12220=EDGE_CURVE('',#9837,#9839,#5255,.T.);
#12221=EDGE_CURVE('',#9840,#9827,#6169,.T.);
#12222=EDGE_CURVE('',#9839,#9840,#6170,.T.);
#12223=EDGE_CURVE('',#9826,#9841,#6171,.T.);
#12224=EDGE_CURVE('',#9840,#9841,#5256,.T.);
#12225=EDGE_CURVE('',#9806,#9842,#6172,.T.);
#12226=EDGE_CURVE('',#9842,#9843,#5257,.T.);
#12227=EDGE_CURVE('',#9843,#9842,#5258,.T.);
#12228=EDGE_CURVE('',#9844,#9844,#5259,.T.);
#12229=EDGE_CURVE('',#9844,#9843,#6173,.T.);
#12230=EDGE_CURVE('',#9845,#9840,#6174,.T.);
#12231=EDGE_CURVE('',#9841,#9846,#6175,.T.);
#12232=EDGE_CURVE('',#9846,#9845,#5260,.T.);
#12233=EDGE_CURVE('',#9847,#9839,#6176,.T.);
#12234=EDGE_CURVE('',#9845,#9847,#6177,.T.);
#12235=EDGE_CURVE('',#9848,#9837,#6178,.T.);
#12236=EDGE_CURVE('',#9847,#9848,#5261,.T.);
#12237=EDGE_CURVE('',#9849,#9838,#6179,.T.);
#12238=EDGE_CURVE('',#9848,#9849,#6180,.T.);
#12239=EDGE_CURVE('',#9850,#9851,#6181,.T.);
#12240=EDGE_CURVE('',#9851,#9838,#5262,.T.);
#12241=EDGE_CURVE('',#9849,#9850,#5263,.T.);
#12242=EDGE_CURVE('',#9852,#9853,#6182,.T.);
#12243=EDGE_CURVE('',#9853,#9851,#6183,.T.);
#12244=EDGE_CURVE('',#9850,#9852,#6184,.T.);
#12245=EDGE_CURVE('',#9854,#9855,#6185,.T.);
#12246=EDGE_CURVE('',#9855,#9853,#5264,.T.);
#12247=EDGE_CURVE('',#9852,#9854,#5265,.T.);
#12248=EDGE_CURVE('',#9841,#9855,#6186,.T.);
#12249=EDGE_CURVE('',#9854,#9846,#6187,.T.);
#12250=EDGE_CURVE('',#9851,#9830,#6188,.T.);
#12251=EDGE_CURVE('',#9853,#9829,#6189,.T.);
#12252=EDGE_CURVE('',#9855,#9828,#6190,.T.);
#12253=EDGE_CURVE('',#9856,#9856,#5266,.T.);
#12254=EDGE_CURVE('',#9857,#9857,#5267,.T.);
#12255=EDGE_CURVE('',#9857,#9858,#6191,.T.);
#12256=EDGE_CURVE('',#9858,#9858,#5268,.T.);
#12257=EDGE_CURVE('',#9859,#9859,#5269,.T.);
#12258=EDGE_CURVE('',#9859,#9857,#6192,.T.);
#12259=EDGE_CURVE('',#9860,#9860,#5270,.T.);
#12260=EDGE_CURVE('',#9860,#9856,#6193,.T.);
#12261=EDGE_CURVE('',#9860,#9861,#6194,.T.);
#12262=EDGE_CURVE('',#9861,#9861,#5271,.T.);
#12263=EDGE_CURVE('',#9861,#9859,#6195,.T.);
#12264=EDGE_CURVE('',#9862,#9863,#6196,.T.);
#12265=EDGE_CURVE('',#9863,#9863,#5272,.T.);
#12266=EDGE_CURVE('',#9863,#9864,#6197,.T.);
#12267=EDGE_CURVE('',#9864,#9864,#5273,.T.);
#12268=EDGE_CURVE('',#9864,#9807,#6198,.T.);
#12269=EDGE_CURVE('',#9865,#9866,#6199,.T.);
#12270=EDGE_CURVE('',#9866,#9866,#5274,.T.);
#12271=EDGE_CURVE('',#9866,#9867,#6200,.T.);
#12272=EDGE_CURVE('',#9867,#9867,#5275,.T.);
#12273=EDGE_CURVE('',#9867,#9808,#6201,.T.);
#12274=EDGE_CURVE('',#9868,#9869,#6202,.T.);
#12275=EDGE_CURVE('',#9869,#9869,#5276,.T.);
#12276=EDGE_CURVE('',#9869,#9870,#6203,.T.);
#12277=EDGE_CURVE('',#9870,#9870,#5277,.T.);
#12278=EDGE_CURVE('',#9870,#9809,#6204,.T.);
#12279=EDGE_CURVE('',#9790,#9815,#6205,.T.);
#12280=EDGE_CURVE('',#9833,#9819,#6206,.T.);
#12281=EDGE_CURVE('',#9820,#9831,#6207,.T.);
#12282=EDGE_CURVE('',#9818,#9835,#6208,.T.);
#15901=ORIENTED_EDGE('',*,*,#12128,.T.);
#15902=ORIENTED_EDGE('',*,*,#12129,.T.);
#15903=ORIENTED_EDGE('',*,*,#12130,.T.);
#15904=ORIENTED_EDGE('',*,*,#12131,.T.);
#15905=ORIENTED_EDGE('',*,*,#12132,.T.);
#15906=ORIENTED_EDGE('',*,*,#12133,.T.);
#15907=ORIENTED_EDGE('',*,*,#12128,.F.);
#15908=ORIENTED_EDGE('',*,*,#12134,.T.);
#15909=ORIENTED_EDGE('',*,*,#12135,.T.);
#15910=ORIENTED_EDGE('',*,*,#12136,.T.);
#15911=ORIENTED_EDGE('',*,*,#12132,.F.);
#15912=ORIENTED_EDGE('',*,*,#12137,.T.);
#15913=ORIENTED_EDGE('',*,*,#12138,.T.);
#15914=ORIENTED_EDGE('',*,*,#12139,.T.);
#15915=ORIENTED_EDGE('',*,*,#12135,.F.);
#15916=ORIENTED_EDGE('',*,*,#12140,.T.);
#15917=ORIENTED_EDGE('',*,*,#12141,.T.);
#15918=ORIENTED_EDGE('',*,*,#12142,.T.);
#15919=ORIENTED_EDGE('',*,*,#12138,.F.);
#15920=ORIENTED_EDGE('',*,*,#12143,.T.);
#15921=ORIENTED_EDGE('',*,*,#12144,.T.);
#15922=ORIENTED_EDGE('',*,*,#12145,.T.);
#15923=ORIENTED_EDGE('',*,*,#12141,.F.);
#15924=ORIENTED_EDGE('',*,*,#12146,.T.);
#15925=ORIENTED_EDGE('',*,*,#12147,.T.);
#15926=ORIENTED_EDGE('',*,*,#12148,.T.);
#15927=ORIENTED_EDGE('',*,*,#12144,.F.);
#15928=ORIENTED_EDGE('',*,*,#12149,.T.);
#15929=ORIENTED_EDGE('',*,*,#12130,.F.);
#15930=ORIENTED_EDGE('',*,*,#12150,.T.);
#15931=ORIENTED_EDGE('',*,*,#12147,.F.);
#15932=ORIENTED_EDGE('',*,*,#12151,.T.);
#15933=ORIENTED_EDGE('',*,*,#12145,.F.);
#15934=ORIENTED_EDGE('',*,*,#12152,.T.);
#15935=ORIENTED_EDGE('',*,*,#12153,.F.);
#15936=ORIENTED_EDGE('',*,*,#12154,.F.);
#15937=ORIENTED_EDGE('',*,*,#12148,.F.);
#15938=ORIENTED_EDGE('',*,*,#12155,.T.);
#15939=ORIENTED_EDGE('',*,*,#12156,.F.);
#15940=ORIENTED_EDGE('',*,*,#12152,.F.);
#15941=ORIENTED_EDGE('',*,*,#12150,.F.);
#15942=ORIENTED_EDGE('',*,*,#12157,.F.);
#15943=ORIENTED_EDGE('',*,*,#12158,.F.);
#15944=ORIENTED_EDGE('',*,*,#12155,.F.);
#15945=ORIENTED_EDGE('',*,*,#12129,.F.);
#15946=ORIENTED_EDGE('',*,*,#12159,.T.);
#15947=ORIENTED_EDGE('',*,*,#12160,.F.);
#15948=ORIENTED_EDGE('',*,*,#12157,.T.);
#15949=ORIENTED_EDGE('',*,*,#12131,.F.);
#15950=ORIENTED_EDGE('',*,*,#12151,.F.);
#15951=ORIENTED_EDGE('',*,*,#12149,.F.);
#15952=ORIENTED_EDGE('',*,*,#12146,.F.);
#15953=ORIENTED_EDGE('',*,*,#12143,.F.);
#15954=ORIENTED_EDGE('',*,*,#12140,.F.);
#15955=ORIENTED_EDGE('',*,*,#12137,.F.);
#15956=ORIENTED_EDGE('',*,*,#12134,.F.);
#15957=ORIENTED_EDGE('',*,*,#12161,.F.);
#15958=ORIENTED_EDGE('',*,*,#12162,.T.);
#15959=ORIENTED_EDGE('',*,*,#12163,.T.);
#15960=ORIENTED_EDGE('',*,*,#12164,.T.);
#15961=ORIENTED_EDGE('',*,*,#12165,.T.);
#15962=ORIENTED_EDGE('',*,*,#12166,.T.);
#15963=ORIENTED_EDGE('',*,*,#12167,.T.);
#15964=ORIENTED_EDGE('',*,*,#12168,.T.);
#15965=ORIENTED_EDGE('',*,*,#12169,.T.);
#15966=ORIENTED_EDGE('',*,*,#12170,.T.);
#15967=ORIENTED_EDGE('',*,*,#12165,.F.);
#15968=ORIENTED_EDGE('',*,*,#12171,.T.);
#15969=ORIENTED_EDGE('',*,*,#12172,.T.);
#15970=ORIENTED_EDGE('',*,*,#12173,.T.);
#15971=ORIENTED_EDGE('',*,*,#12169,.F.);
#15972=ORIENTED_EDGE('',*,*,#12174,.T.);
#15973=ORIENTED_EDGE('',*,*,#12175,.T.);
#15974=ORIENTED_EDGE('',*,*,#12160,.T.);
#15975=ORIENTED_EDGE('',*,*,#12172,.F.);
#15976=ORIENTED_EDGE('',*,*,#12176,.T.);
#15977=ORIENTED_EDGE('',*,*,#12177,.T.);
#15978=ORIENTED_EDGE('',*,*,#12158,.T.);
#15979=ORIENTED_EDGE('',*,*,#12175,.F.);
#15980=ORIENTED_EDGE('',*,*,#12178,.T.);
#15981=ORIENTED_EDGE('',*,*,#12179,.T.);
#15982=ORIENTED_EDGE('',*,*,#12156,.T.);
#15983=ORIENTED_EDGE('',*,*,#12177,.F.);
#15984=ORIENTED_EDGE('',*,*,#12180,.T.);
#15985=ORIENTED_EDGE('',*,*,#12181,.T.);
#15986=ORIENTED_EDGE('',*,*,#12153,.T.);
#15987=ORIENTED_EDGE('',*,*,#12179,.F.);
#15988=ORIENTED_EDGE('',*,*,#12182,.T.);
#15989=ORIENTED_EDGE('',*,*,#12167,.F.);
#15990=ORIENTED_EDGE('',*,*,#12183,.T.);
#15991=ORIENTED_EDGE('',*,*,#12181,.F.);
#15992=ORIENTED_EDGE('',*,*,#12184,.T.);
#15993=ORIENTED_EDGE('',*,*,#12176,.F.);
#15994=ORIENTED_EDGE('',*,*,#12185,.T.);
#15995=ORIENTED_EDGE('',*,*,#12186,.F.);
#15996=ORIENTED_EDGE('',*,*,#12187,.T.);
#15997=ORIENTED_EDGE('',*,*,#12174,.F.);
#15998=ORIENTED_EDGE('',*,*,#12188,.F.);
#15999=ORIENTED_EDGE('',*,*,#12189,.F.);
#16000=ORIENTED_EDGE('',*,*,#12185,.F.);
#16001=ORIENTED_EDGE('',*,*,#12171,.F.);
#16002=ORIENTED_EDGE('',*,*,#12190,.T.);
#16003=ORIENTED_EDGE('',*,*,#12191,.F.);
#16004=ORIENTED_EDGE('',*,*,#12188,.T.);
#16005=ORIENTED_EDGE('',*,*,#12168,.F.);
#16006=ORIENTED_EDGE('',*,*,#12192,.F.);
#16007=ORIENTED_EDGE('',*,*,#12193,.F.);
#16008=ORIENTED_EDGE('',*,*,#12190,.F.);
#16009=ORIENTED_EDGE('',*,*,#12142,.F.);
#16010=ORIENTED_EDGE('',*,*,#12154,.T.);
#16011=ORIENTED_EDGE('',*,*,#12183,.F.);
#16012=ORIENTED_EDGE('',*,*,#12194,.F.);
#16013=ORIENTED_EDGE('',*,*,#12139,.F.);
#16014=ORIENTED_EDGE('',*,*,#12194,.T.);
#16015=ORIENTED_EDGE('',*,*,#12166,.F.);
#16016=ORIENTED_EDGE('',*,*,#12195,.F.);
#16017=ORIENTED_EDGE('',*,*,#12196,.T.);
#16018=ORIENTED_EDGE('',*,*,#12197,.T.);
#16019=ORIENTED_EDGE('',*,*,#12198,.T.);
#16020=ORIENTED_EDGE('',*,*,#12186,.T.);
#16021=ORIENTED_EDGE('',*,*,#12199,.T.);
#16022=ORIENTED_EDGE('',*,*,#12200,.T.);
#16023=ORIENTED_EDGE('',*,*,#12196,.F.);
#16024=ORIENTED_EDGE('',*,*,#12189,.T.);
#16025=ORIENTED_EDGE('',*,*,#12201,.T.);
#16026=ORIENTED_EDGE('',*,*,#12202,.T.);
#16027=ORIENTED_EDGE('',*,*,#12199,.F.);
#16028=ORIENTED_EDGE('',*,*,#12191,.T.);
#16029=ORIENTED_EDGE('',*,*,#12203,.T.);
#16030=ORIENTED_EDGE('',*,*,#12204,.T.);
#16031=ORIENTED_EDGE('',*,*,#12201,.F.);
#16032=ORIENTED_EDGE('',*,*,#12193,.T.);
#16033=ORIENTED_EDGE('',*,*,#12205,.T.);
#16034=ORIENTED_EDGE('',*,*,#12206,.T.);
#16035=ORIENTED_EDGE('',*,*,#12203,.F.);
#16036=ORIENTED_EDGE('',*,*,#12207,.T.);
#16037=ORIENTED_EDGE('',*,*,#12208,.T.);
#16038=ORIENTED_EDGE('',*,*,#12209,.T.);
#16039=ORIENTED_EDGE('',*,*,#12205,.F.);
#16040=ORIENTED_EDGE('',*,*,#12210,.T.);
#16041=ORIENTED_EDGE('',*,*,#12211,.T.);
#16042=ORIENTED_EDGE('',*,*,#12212,.T.);
#16043=ORIENTED_EDGE('',*,*,#12208,.F.);
#16044=ORIENTED_EDGE('',*,*,#12213,.T.);
#16045=ORIENTED_EDGE('',*,*,#12198,.F.);
#16046=ORIENTED_EDGE('',*,*,#12214,.T.);
#16047=ORIENTED_EDGE('',*,*,#12211,.F.);
#16048=ORIENTED_EDGE('',*,*,#12215,.T.);
#16049=ORIENTED_EDGE('',*,*,#12209,.F.);
#16050=ORIENTED_EDGE('',*,*,#12216,.F.);
#16051=ORIENTED_EDGE('',*,*,#12217,.F.);
#16052=ORIENTED_EDGE('',*,*,#12218,.T.);
#16053=ORIENTED_EDGE('',*,*,#12212,.F.);
#16054=ORIENTED_EDGE('',*,*,#12219,.F.);
#16055=ORIENTED_EDGE('',*,*,#12220,.F.);
#16056=ORIENTED_EDGE('',*,*,#12216,.T.);
#16057=ORIENTED_EDGE('',*,*,#12214,.F.);
#16058=ORIENTED_EDGE('',*,*,#12221,.F.);
#16059=ORIENTED_EDGE('',*,*,#12222,.F.);
#16060=ORIENTED_EDGE('',*,*,#12219,.T.);
#16061=ORIENTED_EDGE('',*,*,#12197,.F.);
#16062=ORIENTED_EDGE('',*,*,#12223,.T.);
#16063=ORIENTED_EDGE('',*,*,#12224,.F.);
#16064=ORIENTED_EDGE('',*,*,#12221,.T.);
#16065=ORIENTED_EDGE('',*,*,#12161,.T.);
#16066=ORIENTED_EDGE('',*,*,#12225,.T.);
#16067=ORIENTED_EDGE('',*,*,#12226,.T.);
#16068=ORIENTED_EDGE('',*,*,#12227,.T.);
#16069=ORIENTED_EDGE('',*,*,#12225,.F.);
#16070=ORIENTED_EDGE('',*,*,#12228,.F.);
#16071=ORIENTED_EDGE('',*,*,#12229,.T.);
#16072=ORIENTED_EDGE('',*,*,#12226,.F.);
#16073=ORIENTED_EDGE('',*,*,#12227,.F.);
#16074=ORIENTED_EDGE('',*,*,#12229,.F.);
#16075=ORIENTED_EDGE('',*,*,#12230,.T.);
#16076=ORIENTED_EDGE('',*,*,#12224,.T.);
#16077=ORIENTED_EDGE('',*,*,#12231,.T.);
#16078=ORIENTED_EDGE('',*,*,#12232,.T.);
#16079=ORIENTED_EDGE('',*,*,#12233,.T.);
#16080=ORIENTED_EDGE('',*,*,#12222,.T.);
#16081=ORIENTED_EDGE('',*,*,#12230,.F.);
#16082=ORIENTED_EDGE('',*,*,#12234,.T.);
#16083=ORIENTED_EDGE('',*,*,#12235,.T.);
#16084=ORIENTED_EDGE('',*,*,#12220,.T.);
#16085=ORIENTED_EDGE('',*,*,#12233,.F.);
#16086=ORIENTED_EDGE('',*,*,#12236,.T.);
#16087=ORIENTED_EDGE('',*,*,#12237,.T.);
#16088=ORIENTED_EDGE('',*,*,#12217,.T.);
#16089=ORIENTED_EDGE('',*,*,#12235,.F.);
#16090=ORIENTED_EDGE('',*,*,#12238,.T.);
#16091=ORIENTED_EDGE('',*,*,#12239,.T.);
#16092=ORIENTED_EDGE('',*,*,#12240,.T.);
#16093=ORIENTED_EDGE('',*,*,#12237,.F.);
#16094=ORIENTED_EDGE('',*,*,#12241,.T.);
#16095=ORIENTED_EDGE('',*,*,#12242,.T.);
#16096=ORIENTED_EDGE('',*,*,#12243,.T.);
#16097=ORIENTED_EDGE('',*,*,#12239,.F.);
#16098=ORIENTED_EDGE('',*,*,#12244,.T.);
#16099=ORIENTED_EDGE('',*,*,#12245,.T.);
#16100=ORIENTED_EDGE('',*,*,#12246,.T.);
#16101=ORIENTED_EDGE('',*,*,#12242,.F.);
#16102=ORIENTED_EDGE('',*,*,#12247,.T.);
#16103=ORIENTED_EDGE('',*,*,#12231,.F.);
#16104=ORIENTED_EDGE('',*,*,#12248,.T.);
#16105=ORIENTED_EDGE('',*,*,#12245,.F.);
#16106=ORIENTED_EDGE('',*,*,#12249,.T.);
#16107=ORIENTED_EDGE('',*,*,#12204,.F.);
#16108=ORIENTED_EDGE('',*,*,#12250,.F.);
#16109=ORIENTED_EDGE('',*,*,#12243,.F.);
#16110=ORIENTED_EDGE('',*,*,#12251,.T.);
#16111=ORIENTED_EDGE('',*,*,#12202,.F.);
#16112=ORIENTED_EDGE('',*,*,#12251,.F.);
#16113=ORIENTED_EDGE('',*,*,#12246,.F.);
#16114=ORIENTED_EDGE('',*,*,#12252,.T.);
#16115=ORIENTED_EDGE('',*,*,#12200,.F.);
#16116=ORIENTED_EDGE('',*,*,#12252,.F.);
#16117=ORIENTED_EDGE('',*,*,#12248,.F.);
#16118=ORIENTED_EDGE('',*,*,#12223,.F.);
#16119=ORIENTED_EDGE('',*,*,#12232,.F.);
#16120=ORIENTED_EDGE('',*,*,#12249,.F.);
#16121=ORIENTED_EDGE('',*,*,#12247,.F.);
#16122=ORIENTED_EDGE('',*,*,#12244,.F.);
#16123=ORIENTED_EDGE('',*,*,#12241,.F.);
#16124=ORIENTED_EDGE('',*,*,#12238,.F.);
#16125=ORIENTED_EDGE('',*,*,#12236,.F.);
#16126=ORIENTED_EDGE('',*,*,#12234,.F.);
#16127=ORIENTED_EDGE('',*,*,#12253,.F.);
#16128=ORIENTED_EDGE('',*,*,#12254,.T.);
#16129=ORIENTED_EDGE('',*,*,#12255,.T.);
#16130=ORIENTED_EDGE('',*,*,#12256,.T.);
#16131=ORIENTED_EDGE('',*,*,#12255,.F.);
#16132=ORIENTED_EDGE('',*,*,#12257,.F.);
#16133=ORIENTED_EDGE('',*,*,#12258,.T.);
#16134=ORIENTED_EDGE('',*,*,#12254,.F.);
#16135=ORIENTED_EDGE('',*,*,#12258,.F.);
#16136=ORIENTED_EDGE('',*,*,#12228,.T.);
#16137=ORIENTED_EDGE('',*,*,#12256,.F.);
#16138=ORIENTED_EDGE('',*,*,#12259,.T.);
#16139=ORIENTED_EDGE('',*,*,#12260,.T.);
#16140=ORIENTED_EDGE('',*,*,#12253,.T.);
#16141=ORIENTED_EDGE('',*,*,#12260,.F.);
#16142=ORIENTED_EDGE('',*,*,#12259,.F.);
#16143=ORIENTED_EDGE('',*,*,#12261,.T.);
#16144=ORIENTED_EDGE('',*,*,#12262,.F.);
#16145=ORIENTED_EDGE('',*,*,#12261,.F.);
#16146=ORIENTED_EDGE('',*,*,#12262,.T.);
#16147=ORIENTED_EDGE('',*,*,#12263,.T.);
#16148=ORIENTED_EDGE('',*,*,#12257,.T.);
#16149=ORIENTED_EDGE('',*,*,#12263,.F.);
#16150=ORIENTED_EDGE('',*,*,#12264,.T.);
#16151=ORIENTED_EDGE('',*,*,#12265,.T.);
#16152=ORIENTED_EDGE('',*,*,#12264,.F.);
#16153=ORIENTED_EDGE('',*,*,#12265,.F.);
#16154=ORIENTED_EDGE('',*,*,#12266,.T.);
#16155=ORIENTED_EDGE('',*,*,#12267,.T.);
#16156=ORIENTED_EDGE('',*,*,#12266,.F.);
#16157=ORIENTED_EDGE('',*,*,#12267,.F.);
#16158=ORIENTED_EDGE('',*,*,#12268,.T.);
#16159=ORIENTED_EDGE('',*,*,#12162,.F.);
#16160=ORIENTED_EDGE('',*,*,#12268,.F.);
#16161=ORIENTED_EDGE('',*,*,#12269,.T.);
#16162=ORIENTED_EDGE('',*,*,#12270,.T.);
#16163=ORIENTED_EDGE('',*,*,#12269,.F.);
#16164=ORIENTED_EDGE('',*,*,#12270,.F.);
#16165=ORIENTED_EDGE('',*,*,#12271,.T.);
#16166=ORIENTED_EDGE('',*,*,#12272,.T.);
#16167=ORIENTED_EDGE('',*,*,#12271,.F.);
#16168=ORIENTED_EDGE('',*,*,#12272,.F.);
#16169=ORIENTED_EDGE('',*,*,#12273,.T.);
#16170=ORIENTED_EDGE('',*,*,#12163,.F.);
#16171=ORIENTED_EDGE('',*,*,#12273,.F.);
#16172=ORIENTED_EDGE('',*,*,#12274,.T.);
#16173=ORIENTED_EDGE('',*,*,#12275,.T.);
#16174=ORIENTED_EDGE('',*,*,#12274,.F.);
#16175=ORIENTED_EDGE('',*,*,#12275,.F.);
#16176=ORIENTED_EDGE('',*,*,#12276,.T.);
#16177=ORIENTED_EDGE('',*,*,#12277,.T.);
#16178=ORIENTED_EDGE('',*,*,#12276,.F.);
#16179=ORIENTED_EDGE('',*,*,#12277,.F.);
#16180=ORIENTED_EDGE('',*,*,#12278,.T.);
#16181=ORIENTED_EDGE('',*,*,#12164,.F.);
#16182=ORIENTED_EDGE('',*,*,#12278,.F.);
#16183=ORIENTED_EDGE('',*,*,#12206,.F.);
#16184=ORIENTED_EDGE('',*,*,#12218,.F.);
#16185=ORIENTED_EDGE('',*,*,#12240,.F.);
#16186=ORIENTED_EDGE('',*,*,#12250,.T.);
#16187=ORIENTED_EDGE('',*,*,#12133,.F.);
#16188=ORIENTED_EDGE('',*,*,#12279,.T.);
#16189=ORIENTED_EDGE('',*,*,#12173,.F.);
#16190=ORIENTED_EDGE('',*,*,#12159,.F.);
#16191=ORIENTED_EDGE('',*,*,#12136,.F.);
#16192=ORIENTED_EDGE('',*,*,#12195,.T.);
#16193=ORIENTED_EDGE('',*,*,#12170,.F.);
#16194=ORIENTED_EDGE('',*,*,#12279,.F.);
#16195=ORIENTED_EDGE('',*,*,#12182,.F.);
#16196=ORIENTED_EDGE('',*,*,#12280,.F.);
#16197=ORIENTED_EDGE('',*,*,#12210,.F.);
#16198=ORIENTED_EDGE('',*,*,#12281,.F.);
#16199=ORIENTED_EDGE('',*,*,#12180,.F.);
#16200=ORIENTED_EDGE('',*,*,#12282,.T.);
#16201=ORIENTED_EDGE('',*,*,#12213,.F.);
#16202=ORIENTED_EDGE('',*,*,#12280,.T.);
#16203=ORIENTED_EDGE('',*,*,#12178,.F.);
#16204=ORIENTED_EDGE('',*,*,#12187,.F.);
#16205=ORIENTED_EDGE('',*,*,#12215,.F.);
#16206=ORIENTED_EDGE('',*,*,#12282,.F.);
#16207=ORIENTED_EDGE('',*,*,#12184,.F.);
#16208=ORIENTED_EDGE('',*,*,#12281,.T.);
#16209=ORIENTED_EDGE('',*,*,#12207,.F.);
#16210=ORIENTED_EDGE('',*,*,#12192,.T.);
#21867=CONICAL_SURFACE('',#23857,0.515606601717798,1.17809724509616);
#21868=CONICAL_SURFACE('',#23861,0.515606601717798,1.17809724509617);
#21869=CONICAL_SURFACE('',#23865,0.515606601717798,1.17809724509617);
#21870=CONICAL_SURFACE('',#23869,0.515606601717797,1.17809724509618);
#21871=CONICAL_SURFACE('',#23874,0.56,0.78539816339745);
#21872=CONICAL_SURFACE('',#23877,0.56,0.78539816339745);
#21873=CONICAL_SURFACE('',#23885,0.589393398282202,0.392699081698734);
#21874=CONICAL_SURFACE('',#23889,0.589393398282202,0.392699081698736);
#21875=CONICAL_SURFACE('',#23892,0.589393398282202,0.392699081698712);
#21876=CONICAL_SURFACE('',#23895,0.589393398282202,0.392699081698734);
#21877=CONICAL_SURFACE('',#23904,0.56,0.785398163397448);
#21878=CONICAL_SURFACE('',#23906,0.589393398282202,0.392699081698733);
#21879=CONICAL_SURFACE('',#23909,0.589393398282202,0.392699081698719);
#21880=CONICAL_SURFACE('',#23912,0.589393398282202,0.392699081698719);
#21881=CONICAL_SURFACE('',#23916,0.589393398282202,0.392699081698712);
#21882=CONICAL_SURFACE('',#23921,0.56,0.78539816339745);
#21883=CONICAL_SURFACE('',#23924,0.56,0.78539816339745);
#21884=CONICAL_SURFACE('',#23926,3.79,0.785398163397448);
#21885=CONICAL_SURFACE('',#23931,0.515606601717798,1.17809724509616);
#21886=CONICAL_SURFACE('',#23934,0.515606601717797,1.17809724509619);
#21887=CONICAL_SURFACE('',#23937,0.515606601717798,1.17809724509617);
#21888=CONICAL_SURFACE('',#23941,0.515606601717798,1.17809724509617);
#21889=CONICAL_SURFACE('',#23946,0.56,0.785398163397448);
#21890=CONICAL_SURFACE('',#23950,3.315,0.785398163397448);
#21891=CONICAL_SURFACE('',#23956,3.3543933982822,1.17809724509617);
#21892=CONICAL_SURFACE('',#23958,3.325,0.785398163397446);
#21893=CONICAL_SURFACE('',#23960,3.3106066017178,0.392699081698723);
#21894=CONICAL_SURFACE('',#23961,0.1025,1.02974425867666);
#21895=CONICAL_SURFACE('',#23965,0.255,0.785398163397448);
#21896=CONICAL_SURFACE('',#23966,0.1025,1.02974425867666);
#21897=CONICAL_SURFACE('',#23970,0.255,0.785398163397446);
#21898=CONICAL_SURFACE('',#23971,0.1025,1.02974425867666);
#21899=CONICAL_SURFACE('',#23975,0.255,0.785398163397446);
#21900=CONICAL_SURFACE('',#23976,0.56,0.785398163397448);
#21901=CONICAL_SURFACE('',#23978,0.56,0.785398163397448);
#22168=ADVANCED_FACE('',(#2429),#21867,.T.);
#22169=ADVANCED_FACE('',(#2430),#1518,.T.);
#22170=ADVANCED_FACE('',(#2431),#21868,.T.);
#22171=ADVANCED_FACE('',(#2432),#1519,.T.);
#22172=ADVANCED_FACE('',(#2433),#21869,.T.);
#22173=ADVANCED_FACE('',(#2434),#1520,.T.);
#22174=ADVANCED_FACE('',(#2435),#21870,.T.);
#22175=ADVANCED_FACE('',(#2436),#1521,.T.);
#22176=ADVANCED_FACE('',(#2437),#1522,.T.);
#22177=ADVANCED_FACE('',(#2438),#21871,.T.);
#22178=ADVANCED_FACE('',(#2439),#1523,.T.);
#22179=ADVANCED_FACE('',(#2440),#21872,.T.);
#22180=ADVANCED_FACE('',(#2441,#1320,#1321,#1322,#1323),#1524,.F.);
#22181=ADVANCED_FACE('',(#2442),#1525,.T.);
#22182=ADVANCED_FACE('',(#2443),#21873,.T.);
#22183=ADVANCED_FACE('',(#2444),#1526,.T.);
#22184=ADVANCED_FACE('',(#2445),#21874,.T.);
#22185=ADVANCED_FACE('',(#2446),#1527,.T.);
#22186=ADVANCED_FACE('',(#2447),#21875,.T.);
#22187=ADVANCED_FACE('',(#2448),#1528,.T.);
#22188=ADVANCED_FACE('',(#2449),#21876,.T.);
#22189=ADVANCED_FACE('',(#2450),#978,.T.);
#22190=ADVANCED_FACE('',(#2451),#1529,.T.);
#22191=ADVANCED_FACE('',(#2452),#979,.T.);
#22192=ADVANCED_FACE('',(#2453),#1530,.T.);
#22193=ADVANCED_FACE('',(#2454),#21877,.T.);
#22194=ADVANCED_FACE('',(#2455),#1531,.T.);
#22195=ADVANCED_FACE('',(#2456),#21878,.T.);
#22196=ADVANCED_FACE('',(#2457),#1532,.T.);
#22197=ADVANCED_FACE('',(#2458),#21879,.T.);
#22198=ADVANCED_FACE('',(#2459),#1533,.T.);
#22199=ADVANCED_FACE('',(#2460),#21880,.T.);
#22200=ADVANCED_FACE('',(#2461),#1534,.T.);
#22201=ADVANCED_FACE('',(#2462),#21881,.T.);
#22202=ADVANCED_FACE('',(#2463),#1535,.T.);
#22203=ADVANCED_FACE('',(#2464),#1536,.T.);
#22204=ADVANCED_FACE('',(#2465),#21882,.T.);
#22205=ADVANCED_FACE('',(#2466),#1537,.T.);
#22206=ADVANCED_FACE('',(#2467),#21883,.T.);
#22207=ADVANCED_FACE('',(#2468),#21884,.F.);
#22208=ADVANCED_FACE('',(#2469),#980,.F.);
#22209=ADVANCED_FACE('',(#2470),#21885,.T.);
#22210=ADVANCED_FACE('',(#2471),#1538,.T.);
#22211=ADVANCED_FACE('',(#2472),#21886,.T.);
#22212=ADVANCED_FACE('',(#2473),#1539,.T.);
#22213=ADVANCED_FACE('',(#2474),#21887,.T.);
#22214=ADVANCED_FACE('',(#2475),#1540,.T.);
#22215=ADVANCED_FACE('',(#2476),#21888,.T.);
#22216=ADVANCED_FACE('',(#2477),#1541,.T.);
#22217=ADVANCED_FACE('',(#2478),#1542,.T.);
#22218=ADVANCED_FACE('',(#2479),#21889,.T.);
#22219=ADVANCED_FACE('',(#2480),#1543,.T.);
#22220=ADVANCED_FACE('',(#2481,#1324),#1544,.T.);
#22221=ADVANCED_FACE('',(#2482),#21890,.F.);
#22222=ADVANCED_FACE('',(#2483),#981,.F.);
#22223=ADVANCED_FACE('',(#2484,#1325),#1545,.F.);
#22224=ADVANCED_FACE('',(#2485),#21891,.F.);
#22225=ADVANCED_FACE('',(#2486),#21892,.F.);
#22226=ADVANCED_FACE('',(#2487),#21893,.F.);
#22227=ADVANCED_FACE('',(#2488),#21894,.F.);
#22228=ADVANCED_FACE('',(#2489),#982,.F.);
#22229=ADVANCED_FACE('',(#2490),#21895,.F.);
#22230=ADVANCED_FACE('',(#2491),#21896,.F.);
#22231=ADVANCED_FACE('',(#2492),#983,.F.);
#22232=ADVANCED_FACE('',(#2493),#21897,.F.);
#22233=ADVANCED_FACE('',(#2494),#21898,.F.);
#22234=ADVANCED_FACE('',(#2495),#984,.F.);
#22235=ADVANCED_FACE('',(#2496),#21899,.F.);
#22236=ADVANCED_FACE('',(#2497),#21900,.T.);
#22237=ADVANCED_FACE('',(#2498),#1546,.T.);
#22238=ADVANCED_FACE('',(#2499),#21901,.T.);
#22239=ADVANCED_FACE('',(#2500),#1547,.T.);
#22240=ADVANCED_FACE('',(#2501),#985,.T.);
#22241=ADVANCED_FACE('',(#2502),#1548,.T.);
#22242=ADVANCED_FACE('',(#2503),#986,.T.);
#23305=CLOSED_SHELL('',(#22168,#22169,#22170,#22171,#22172,#22173,#22174,
#22175,#22176,#22177,#22178,#22179,#22180,#22181,#22182,#22183,#22184,#22185,
#22186,#22187,#22188,#22189,#22190,#22191,#22192,#22193,#22194,#22195,#22196,
#22197,#22198,#22199,#22200,#22201,#22202,#22203,#22204,#22205,#22206,#22207,
#22208,#22209,#22210,#22211,#22212,#22213,#22214,#22215,#22216,#22217,#22218,
#22219,#22220,#22221,#22222,#22223,#22224,#22225,#22226,#22227,#22228,#22229,
#22230,#22231,#22232,#22233,#22234,#22235,#22236,#22237,#22238,#22239,#22240,
#22241,#22242));
#23856=AXIS2_PLACEMENT_3D('',#32671,#26627,#26628);
#23857=AXIS2_PLACEMENT_3D('',#32672,#26629,#26630);
#23858=AXIS2_PLACEMENT_3D('',#32677,#26632,#26633);
#23859=AXIS2_PLACEMENT_3D('',#32680,#26635,#26636);
#23860=AXIS2_PLACEMENT_3D('',#32681,#26637,#26638);
#23861=AXIS2_PLACEMENT_3D('',#32687,#26642,#26643);
#23862=AXIS2_PLACEMENT_3D('',#32691,#26645,#26646);
#23863=AXIS2_PLACEMENT_3D('',#32692,#26647,#26648);
#23864=AXIS2_PLACEMENT_3D('',#32693,#26649,#26650);
#23865=AXIS2_PLACEMENT_3D('',#32699,#26654,#26655);
#23866=AXIS2_PLACEMENT_3D('',#32703,#26657,#26658);
#23867=AXIS2_PLACEMENT_3D('',#32704,#26659,#26660);
#23868=AXIS2_PLACEMENT_3D('',#32705,#26661,#26662);
#23869=AXIS2_PLACEMENT_3D('',#32711,#26666,#26667);
#23870=AXIS2_PLACEMENT_3D('',#32715,#26669,#26670);
#23871=AXIS2_PLACEMENT_3D('',#32716,#26671,#26672);
#23872=AXIS2_PLACEMENT_3D('',#32717,#26673,#26674);
#23873=AXIS2_PLACEMENT_3D('',#32720,#26677,#26678);
#23874=AXIS2_PLACEMENT_3D('',#32726,#26682,#26683);
#23875=AXIS2_PLACEMENT_3D('',#32729,#26685,#26686);
#23876=AXIS2_PLACEMENT_3D('',#32730,#26687,#26688);
#23877=AXIS2_PLACEMENT_3D('',#32734,#26691,#26692);
#23878=AXIS2_PLACEMENT_3D('',#32737,#26694,#26695);
#23879=AXIS2_PLACEMENT_3D('',#32738,#26696,#26697);
#23880=AXIS2_PLACEMENT_3D('',#32740,#26698,#26699);
#23881=AXIS2_PLACEMENT_3D('',#32742,#26700,#26701);
#23882=AXIS2_PLACEMENT_3D('',#32744,#26702,#26703);
#23883=AXIS2_PLACEMENT_3D('',#32746,#26704,#26705);
#23884=AXIS2_PLACEMENT_3D('',#32747,#26706,#26707);
#23885=AXIS2_PLACEMENT_3D('',#32756,#26712,#26713);
#23886=AXIS2_PLACEMENT_3D('',#32760,#26715,#26716);
#23887=AXIS2_PLACEMENT_3D('',#32761,#26717,#26718);
#23888=AXIS2_PLACEMENT_3D('',#32762,#26719,#26720);
#23889=AXIS2_PLACEMENT_3D('',#32767,#26724,#26725);
#23890=AXIS2_PLACEMENT_3D('',#32770,#26727,#26728);
#23891=AXIS2_PLACEMENT_3D('',#32771,#26729,#26730);
#23892=AXIS2_PLACEMENT_3D('',#32775,#26733,#26734);
#23893=AXIS2_PLACEMENT_3D('',#32778,#26736,#26737);
#23894=AXIS2_PLACEMENT_3D('',#32779,#26738,#26739);
#23895=AXIS2_PLACEMENT_3D('',#32783,#26742,#26743);
#23896=AXIS2_PLACEMENT_3D('',#32784,#26744,#26745);
#23897=AXIS2_PLACEMENT_3D('',#32785,#26746,#26747);
#23898=AXIS2_PLACEMENT_3D('',#32786,#26748,#26749);
#23899=AXIS2_PLACEMENT_3D('',#32790,#26751,#26752);
#23900=AXIS2_PLACEMENT_3D('',#32792,#26754,#26755);
#23901=AXIS2_PLACEMENT_3D('',#32796,#26758,#26759);
#23902=AXIS2_PLACEMENT_3D('',#32799,#26761,#26762);
#23903=AXIS2_PLACEMENT_3D('',#32800,#26763,#26764);
#23904=AXIS2_PLACEMENT_3D('',#32804,#26767,#26768);
#23905=AXIS2_PLACEMENT_3D('',#32806,#26770,#26771);
#23906=AXIS2_PLACEMENT_3D('',#32808,#26773,#26774);
#23907=AXIS2_PLACEMENT_3D('',#32812,#26776,#26777);
#23908=AXIS2_PLACEMENT_3D('',#32814,#26779,#26780);
#23909=AXIS2_PLACEMENT_3D('',#32818,#26783,#26784);
#23910=AXIS2_PLACEMENT_3D('',#32821,#26786,#26787);
#23911=AXIS2_PLACEMENT_3D('',#32822,#26788,#26789);
#23912=AXIS2_PLACEMENT_3D('',#32826,#26792,#26793);
#23913=AXIS2_PLACEMENT_3D('',#32830,#26795,#26796);
#23914=AXIS2_PLACEMENT_3D('',#32831,#26797,#26798);
#23915=AXIS2_PLACEMENT_3D('',#32832,#26799,#26800);
#23916=AXIS2_PLACEMENT_3D('',#32838,#26804,#26805);
#23917=AXIS2_PLACEMENT_3D('',#32842,#26807,#26808);
#23918=AXIS2_PLACEMENT_3D('',#32843,#26809,#26810);
#23919=AXIS2_PLACEMENT_3D('',#32844,#26811,#26812);
#23920=AXIS2_PLACEMENT_3D('',#32847,#26815,#26816);
#23921=AXIS2_PLACEMENT_3D('',#32853,#26820,#26821);
#23922=AXIS2_PLACEMENT_3D('',#32856,#26823,#26824);
#23923=AXIS2_PLACEMENT_3D('',#32857,#26825,#26826);
#23924=AXIS2_PLACEMENT_3D('',#32861,#26829,#26830);
#23925=AXIS2_PLACEMENT_3D('',#32864,#26832,#26833);
#23926=AXIS2_PLACEMENT_3D('',#32865,#26834,#26835);
#23927=AXIS2_PLACEMENT_3D('',#32869,#26837,#26838);
#23928=AXIS2_PLACEMENT_3D('',#32870,#26839,#26840);
#23929=AXIS2_PLACEMENT_3D('',#32871,#26841,#26842);
#23930=AXIS2_PLACEMENT_3D('',#32873,#26843,#26844);
#23931=AXIS2_PLACEMENT_3D('',#32875,#26846,#26847);
#23932=AXIS2_PLACEMENT_3D('',#32880,#26850,#26851);
#23933=AXIS2_PLACEMENT_3D('',#32881,#26852,#26853);
#23934=AXIS2_PLACEMENT_3D('',#32885,#26856,#26857);
#23935=AXIS2_PLACEMENT_3D('',#32888,#26859,#26860);
#23936=AXIS2_PLACEMENT_3D('',#32889,#26861,#26862);
#23937=AXIS2_PLACEMENT_3D('',#32893,#26865,#26866);
#23938=AXIS2_PLACEMENT_3D('',#32897,#26868,#26869);
#23939=AXIS2_PLACEMENT_3D('',#32898,#26870,#26871);
#23940=AXIS2_PLACEMENT_3D('',#32899,#26872,#26873);
#23941=AXIS2_PLACEMENT_3D('',#32905,#26877,#26878);
#23942=AXIS2_PLACEMENT_3D('',#32909,#26880,#26881);
#23943=AXIS2_PLACEMENT_3D('',#32910,#26882,#26883);
#23944=AXIS2_PLACEMENT_3D('',#32911,#26884,#26885);
#23945=AXIS2_PLACEMENT_3D('',#32914,#26888,#26889);
#23946=AXIS2_PLACEMENT_3D('',#32917,#26892,#26893);
#23947=AXIS2_PLACEMENT_3D('',#32919,#26895,#26896);
#23948=AXIS2_PLACEMENT_3D('',#32920,#26897,#26898);
#23949=AXIS2_PLACEMENT_3D('',#32922,#26899,#26900);
#23950=AXIS2_PLACEMENT_3D('',#32923,#26901,#26902);
#23951=AXIS2_PLACEMENT_3D('',#32925,#26903,#26904);
#23952=AXIS2_PLACEMENT_3D('',#32928,#26906,#26907);
#23953=AXIS2_PLACEMENT_3D('',#32929,#26908,#26909);
#23954=AXIS2_PLACEMENT_3D('',#32931,#26910,#26911);
#23955=AXIS2_PLACEMENT_3D('',#32933,#26913,#26914);
#23956=AXIS2_PLACEMENT_3D('',#32934,#26915,#26916);
#23957=AXIS2_PLACEMENT_3D('',#32936,#26917,#26918);
#23958=AXIS2_PLACEMENT_3D('',#32938,#26920,#26921);
#23959=AXIS2_PLACEMENT_3D('',#32941,#26923,#26924);
#23960=AXIS2_PLACEMENT_3D('',#32942,#26925,#26926);
#23961=AXIS2_PLACEMENT_3D('',#32944,#26928,#26929);
#23962=AXIS2_PLACEMENT_3D('',#32948,#26931,#26932);
#23963=AXIS2_PLACEMENT_3D('',#32949,#26933,#26934);
#23964=AXIS2_PLACEMENT_3D('',#32952,#26936,#26937);
#23965=AXIS2_PLACEMENT_3D('',#32953,#26938,#26939);
#23966=AXIS2_PLACEMENT_3D('',#32955,#26941,#26942);
#23967=AXIS2_PLACEMENT_3D('',#32959,#26944,#26945);
#23968=AXIS2_PLACEMENT_3D('',#32960,#26946,#26947);
#23969=AXIS2_PLACEMENT_3D('',#32963,#26949,#26950);
#23970=AXIS2_PLACEMENT_3D('',#32964,#26951,#26952);
#23971=AXIS2_PLACEMENT_3D('',#32966,#26954,#26955);
#23972=AXIS2_PLACEMENT_3D('',#32970,#26957,#26958);
#23973=AXIS2_PLACEMENT_3D('',#32971,#26959,#26960);
#23974=AXIS2_PLACEMENT_3D('',#32974,#26962,#26963);
#23975=AXIS2_PLACEMENT_3D('',#32975,#26964,#26965);
#23976=AXIS2_PLACEMENT_3D('',#32977,#26967,#26968);
#23977=AXIS2_PLACEMENT_3D('',#32978,#26969,#26970);
#23978=AXIS2_PLACEMENT_3D('',#32980,#26972,#26973);
#23979=AXIS2_PLACEMENT_3D('',#32981,#26974,#26975);
#23980=AXIS2_PLACEMENT_3D('',#32984,#26978,#26979);
#23981=AXIS2_PLACEMENT_3D('',#32986,#26981,#26982);
#23982=AXIS2_PLACEMENT_3D('',#32987,#26983,#26984);
#26627=DIRECTION('axis',(0.,0.,1.));
#26628=DIRECTION('refdir',(1.,0.,0.));
#26629=DIRECTION('center_axis',(0.,1.,0.));
#26630=DIRECTION('ref_axis',(0.707106781186546,0.,0.707106781186549));
#26631=DIRECTION('',(0.923879532511281,0.382683432365105,0.));
#26632=DIRECTION('center_axis',(-1.16042435677245E-15,-1.,1.16042435677245E-15));
#26633=DIRECTION('ref_axis',(0.707106781186546,0.,0.707106781186549));
#26634=DIRECTION('',(1.60226232325242E-14,-0.382683432365069,-0.923879532511295));
#26635=DIRECTION('center_axis',(0.,1.,0.));
#26636=DIRECTION('ref_axis',(0.707106781186546,0.,0.707106781186549));
#26637=DIRECTION('center_axis',(0.382683432365084,-0.923879532511289,0.));
#26638=DIRECTION('ref_axis',(0.,0.,-1.));
#26639=DIRECTION('',(0.923879532511289,0.382683432365084,0.));
#26640=DIRECTION('',(0.,0.,1.));
#26641=DIRECTION('',(0.,0.,-1.));
#26642=DIRECTION('center_axis',(0.,1.,0.));
#26643=DIRECTION('ref_axis',(0.707106781186548,0.,-0.707106781186547));
#26644=DIRECTION('',(0.,0.382683432365101,-0.923879532511282));
#26645=DIRECTION('center_axis',(0.,-1.,0.));
#26646=DIRECTION('ref_axis',(0.707106781186548,0.,-0.707106781186547));
#26647=DIRECTION('center_axis',(0.,1.,0.));
#26648=DIRECTION('ref_axis',(0.707106781186548,0.,-0.707106781186548));
#26649=DIRECTION('center_axis',(0.,-0.923879532511291,-0.38268343236508));
#26650=DIRECTION('ref_axis',(0.,0.38268343236508,-0.923879532511291));
#26651=DIRECTION('',(0.,0.38268343236509,-0.923879532511287));
#26652=DIRECTION('',(1.,0.,0.));
#26653=DIRECTION('',(-1.,0.,0.));
#26654=DIRECTION('center_axis',(0.,1.,0.));
#26655=DIRECTION('ref_axis',(-0.707106781186548,0.,-0.707106781186547));
#26656=DIRECTION('',(-0.923879532511284,0.382683432365097,0.));
#26657=DIRECTION('center_axis',(0.,-1.,0.));
#26658=DIRECTION('ref_axis',(-0.707106781186548,0.,-0.707106781186547));
#26659=DIRECTION('center_axis',(0.,1.,0.));
#26660=DIRECTION('ref_axis',(-0.707106781186548,0.,-0.707106781186548));
#26661=DIRECTION('center_axis',(-0.382683432365084,-0.923879532511289,0.));
#26662=DIRECTION('ref_axis',(0.,0.,-1.));
#26663=DIRECTION('',(-0.923879532511289,0.382683432365084,0.));
#26664=DIRECTION('',(0.,0.,-1.));
#26665=DIRECTION('',(0.,0.,1.));
#26666=DIRECTION('center_axis',(0.,1.,0.));
#26667=DIRECTION('ref_axis',(-0.707106781186549,0.,0.707106781186547));
#26668=DIRECTION('',(0.,0.382683432365085,0.923879532511289));
#26669=DIRECTION('center_axis',(0.,-1.,0.));
#26670=DIRECTION('ref_axis',(-0.707106781186548,0.,0.707106781186547));
#26671=DIRECTION('center_axis',(0.,1.,0.));
#26672=DIRECTION('ref_axis',(-0.707106781186548,0.,0.707106781186547));
#26673=DIRECTION('center_axis',(0.,-0.92387953251129,0.382683432365083));
#26674=DIRECTION('ref_axis',(0.,-0.382683432365083,-0.92387953251129));
#26675=DIRECTION('',(-1.,0.,0.));
#26676=DIRECTION('',(1.,0.,0.));
#26677=DIRECTION('center_axis',(-0.707106781186548,-0.707106781186548,0.));
#26678=DIRECTION('ref_axis',(0.,0.,1.));
#26679=DIRECTION('',(-0.707106781186548,0.707106781186548,0.));
#26680=DIRECTION('',(0.,0.,1.));
#26681=DIRECTION('',(-0.707106781186548,0.707106781186548,0.));
#26682=DIRECTION('center_axis',(0.,1.,0.));
#26683=DIRECTION('ref_axis',(-0.707106781186548,0.,0.707106781186546));
#26684=DIRECTION('',(0.,0.707106781186548,0.707106781186548));
#26685=DIRECTION('center_axis',(0.,1.,0.));
#26686=DIRECTION('ref_axis',(-0.707106781186547,0.,0.707106781186547));
#26687=DIRECTION('center_axis',(0.,-0.707106781186548,0.707106781186548));
#26688=DIRECTION('ref_axis',(1.,0.,0.));
#26689=DIRECTION('',(0.,-0.707106781186548,-0.707106781186548));
#26690=DIRECTION('',(1.,0.,0.));
#26691=DIRECTION('center_axis',(0.,1.,0.));
#26692=DIRECTION('ref_axis',(0.707106781186546,0.,0.707106781186549));
#26693=DIRECTION('',(0.707106781186548,0.707106781186548,0.));
#26694=DIRECTION('center_axis',(-1.62763815761205E-15,1.,1.62763815761205E-15));
#26695=DIRECTION('ref_axis',(0.707106781186547,0.,0.707106781186548));
#26696=DIRECTION('center_axis',(0.,1.,0.));
#26697=DIRECTION('ref_axis',(1.,0.,0.));
#26698=DIRECTION('center_axis',(0.,-1.,0.));
#26699=DIRECTION('ref_axis',(-1.,0.,0.));
#26700=DIRECTION('center_axis',(0.,1.,0.));
#26701=DIRECTION('ref_axis',(1.,0.,0.));
#26702=DIRECTION('center_axis',(0.,1.,0.));
#26703=DIRECTION('ref_axis',(1.,0.,0.));
#26704=DIRECTION('center_axis',(0.,1.,0.));
#26705=DIRECTION('ref_axis',(1.,0.,0.));
#26706=DIRECTION('center_axis',(0.,-0.382683432365099,-0.923879532511283));
#26707=DIRECTION('ref_axis',(-1.,0.,0.));
#26708=DIRECTION('',(0.,-0.923879532511286,0.382683432365093));
#26709=DIRECTION('',(-1.,0.,0.));
#26710=DIRECTION('',(0.,0.923879532511286,-0.382683432365093));
#26711=DIRECTION('',(1.,0.,0.));
#26712=DIRECTION('center_axis',(0.,1.,0.));
#26713=DIRECTION('ref_axis',(0.707106781186547,0.,-0.707106781186548));
#26714=DIRECTION('',(-0.382683432365089,-0.923879532511287,0.));
#26715=DIRECTION('center_axis',(0.,1.,0.));
#26716=DIRECTION('ref_axis',(0.707106781186547,0.,-0.707106781186548));
#26717=DIRECTION('center_axis',(0.,-1.,0.));
#26718=DIRECTION('ref_axis',(0.707106781186547,0.,-0.707106781186547));
#26719=DIRECTION('center_axis',(0.923879532511284,-0.382683432365097,0.));
#26720=DIRECTION('ref_axis',(0.,0.,-1.));
#26721=DIRECTION('',(-0.382683432365097,-0.923879532511284,0.));
#26722=DIRECTION('',(0.,0.,-1.));
#26723=DIRECTION('',(0.,0.,1.));
#26724=DIRECTION('center_axis',(0.,1.,0.));
#26725=DIRECTION('ref_axis',(0.707106781186547,0.,0.707106781186549));
#26726=DIRECTION('',(-1.60226232325235E-14,-0.923879532511276,-0.382683432365116));
#26727=DIRECTION('center_axis',(0.,-1.,0.));
#26728=DIRECTION('ref_axis',(0.707106781186546,0.,0.707106781186549));
#26729=DIRECTION('center_axis',(0.,-0.382683432365088,0.923879532511288));
#26730=DIRECTION('ref_axis',(1.,0.,0.));
#26731=DIRECTION('',(0.,-0.923879532511285,-0.382683432365094));
#26732=DIRECTION('',(-1.,0.,0.));
#26733=DIRECTION('center_axis',(0.,1.,0.));
#26734=DIRECTION('ref_axis',(-0.707106781186548,0.,0.707106781186547));
#26735=DIRECTION('',(0.382683432365083,-0.92387953251129,0.));
#26736=DIRECTION('center_axis',(0.,-1.,0.));
#26737=DIRECTION('ref_axis',(-0.707106781186548,0.,0.707106781186546));
#26738=DIRECTION('center_axis',(-0.923879532511284,-0.382683432365097,0.));
#26739=DIRECTION('ref_axis',(0.,0.,1.));
#26740=DIRECTION('',(0.382683432365097,-0.923879532511284,0.));
#26741=DIRECTION('',(0.,0.,-1.));
#26742=DIRECTION('center_axis',(0.,1.,0.));
#26743=DIRECTION('ref_axis',(-0.707106781186547,0.,-0.707106781186548));
#26744=DIRECTION('center_axis',(0.,1.,0.));
#26745=DIRECTION('ref_axis',(-0.707106781186547,0.,-0.707106781186548));
#26746=DIRECTION('center_axis',(0.,-1.,0.));
#26747=DIRECTION('ref_axis',(-0.707106781186547,0.,-0.707106781186547));
#26748=DIRECTION('center_axis',(0.,1.,0.));
#26749=DIRECTION('ref_axis',(0.707106781186546,0.,0.707106781186549));
#26750=DIRECTION('',(0.,1.,0.));
#26751=DIRECTION('center_axis',(0.,1.,0.));
#26752=DIRECTION('ref_axis',(0.707106781186546,0.,0.707106781186549));
#26753=DIRECTION('',(0.,-1.,0.));
#26754=DIRECTION('center_axis',(1.,0.,0.));
#26755=DIRECTION('ref_axis',(0.,0.,-1.));
#26756=DIRECTION('',(0.,-1.,0.));
#26757=DIRECTION('',(0.,0.,-1.));
#26758=DIRECTION('center_axis',(0.,1.,0.));
#26759=DIRECTION('ref_axis',(0.707106781186547,0.,-0.707106781186547));
#26760=DIRECTION('',(0.,1.,0.));
#26761=DIRECTION('center_axis',(0.,1.,0.));
#26762=DIRECTION('ref_axis',(0.707106781186547,0.,-0.707106781186547));
#26763=DIRECTION('center_axis',(0.,0.,-1.));
#26764=DIRECTION('ref_axis',(-1.,0.,0.));
#26765=DIRECTION('',(0.,-1.,0.));
#26766=DIRECTION('',(-1.,0.,0.));
#26767=DIRECTION('center_axis',(0.,1.,0.));
#26768=DIRECTION('ref_axis',(-0.707106781186548,0.,-0.707106781186548));
#26769=DIRECTION('',(0.,0.707106781186548,-0.707106781186548));
#26770=DIRECTION('center_axis',(0.,-0.707106781186548,-0.707106781186548));
#26771=DIRECTION('ref_axis',(-1.,0.,0.));
#26772=DIRECTION('',(0.,0.707106781186548,-0.707106781186548));
#26773=DIRECTION('center_axis',(0.,-1.,0.));
#26774=DIRECTION('ref_axis',(0.707106781186547,0.,0.707106781186549));
#26775=DIRECTION('',(-0.382683432365089,0.923879532511287,0.));
#26776=DIRECTION('center_axis',(1.0850921050747E-15,-1.,-1.0850921050747E-15));
#26777=DIRECTION('ref_axis',(0.707106781186547,0.,0.707106781186548));
#26778=DIRECTION('',(1.60226232325234E-14,-0.923879532511277,0.382683432365113));
#26779=DIRECTION('center_axis',(0.923879532511286,0.382683432365092,0.));
#26780=DIRECTION('ref_axis',(0.,0.,-1.));
#26781=DIRECTION('',(-0.382683432365092,0.923879532511286,0.));
#26782=DIRECTION('',(0.,0.,1.));
#26783=DIRECTION('center_axis',(0.,-1.,0.));
#26784=DIRECTION('ref_axis',(0.707106781186547,0.,-0.707106781186547));
#26785=DIRECTION('',(0.,0.92387953251129,0.382683432365082));
#26786=DIRECTION('center_axis',(0.,-1.,0.));
#26787=DIRECTION('ref_axis',(0.707106781186547,0.,-0.707106781186547));
#26788=DIRECTION('center_axis',(0.,0.382683432365088,-0.923879532511287));
#26789=DIRECTION('ref_axis',(-1.,0.,0.));
#26790=DIRECTION('',(0.,0.923879532511287,0.382683432365088));
#26791=DIRECTION('',(1.,0.,0.));
#26792=DIRECTION('center_axis',(0.,-1.,0.));
#26793=DIRECTION('ref_axis',(-0.707106781186547,0.,-0.707106781186547));
#26794=DIRECTION('',(0.382683432365086,0.923879532511288,0.));
#26795=DIRECTION('center_axis',(0.,-1.,0.));
#26796=DIRECTION('ref_axis',(-0.707106781186547,0.,-0.707106781186547));
#26797=DIRECTION('center_axis',(0.,1.,0.));
#26798=DIRECTION('ref_axis',(-0.707106781186547,0.,-0.707106781186547));
#26799=DIRECTION('center_axis',(-0.923879532511286,0.382683432365092,0.));
#26800=DIRECTION('ref_axis',(0.,0.,1.));
#26801=DIRECTION('',(0.382683432365092,0.923879532511286,0.));
#26802=DIRECTION('',(0.,0.,-1.));
#26803=DIRECTION('',(0.,0.,1.));
#26804=DIRECTION('center_axis',(0.,-1.,0.));
#26805=DIRECTION('ref_axis',(-0.707106781186548,0.,0.707106781186547));
#26806=DIRECTION('',(0.,0.923879532511294,-0.382683432365072));
#26807=DIRECTION('center_axis',(0.,-1.,0.));
#26808=DIRECTION('ref_axis',(-0.707106781186547,0.,0.707106781186547));
#26809=DIRECTION('center_axis',(0.,1.,0.));
#26810=DIRECTION('ref_axis',(-0.707106781186548,0.,0.707106781186546));
#26811=DIRECTION('center_axis',(0.,0.382683432365087,0.923879532511288));
#26812=DIRECTION('ref_axis',(1.,0.,0.));
#26813=DIRECTION('',(-1.,0.,0.));
#26814=DIRECTION('',(1.,0.,0.));
#26815=DIRECTION('center_axis',(-0.707106781186549,0.707106781186547,0.));
#26816=DIRECTION('ref_axis',(0.,0.,1.));
#26817=DIRECTION('',(-0.707106781186548,-0.707106781186548,0.));
#26818=DIRECTION('',(0.,0.,1.));
#26819=DIRECTION('',(-0.707106781186547,-0.707106781186549,0.));
#26820=DIRECTION('center_axis',(0.,-1.,0.));
#26821=DIRECTION('ref_axis',(-0.707106781186548,0.,0.707106781186546));
#26822=DIRECTION('',(0.,-0.707106781186549,0.707106781186547));
#26823=DIRECTION('center_axis',(0.,1.,0.));
#26824=DIRECTION('ref_axis',(-0.707106781186548,0.,0.707106781186547));
#26825=DIRECTION('center_axis',(0.,0.707106781186547,0.707106781186549));
#26826=DIRECTION('ref_axis',(1.,0.,0.));
#26827=DIRECTION('',(0.,-0.707106781186548,0.707106781186548));
#26828=DIRECTION('',(1.,0.,0.));
#26829=DIRECTION('center_axis',(0.,-1.,0.));
#26830=DIRECTION('ref_axis',(0.707106781186546,0.,0.707106781186549));
#26831=DIRECTION('',(-0.707106781186548,0.707106781186548,0.));
#26832=DIRECTION('center_axis',(0.,1.,0.));
#26833=DIRECTION('ref_axis',(0.707106781186546,0.,0.707106781186549));
#26834=DIRECTION('center_axis',(0.,-1.,0.));
#26835=DIRECTION('ref_axis',(-1.,0.,0.));
#26836=DIRECTION('',(-0.707106781186548,0.707106781186548,-8.65956056235493E-17));
#26837=DIRECTION('center_axis',(0.,1.,0.));
#26838=DIRECTION('ref_axis',(-1.,0.,0.));
#26839=DIRECTION('center_axis',(0.,1.,0.));
#26840=DIRECTION('ref_axis',(-1.,0.,0.));
#26841=DIRECTION('center_axis',(0.,-1.,0.));
#26842=DIRECTION('ref_axis',(1.,0.,0.));
#26843=DIRECTION('center_axis',(0.,-1.,0.));
#26844=DIRECTION('ref_axis',(1.,0.,0.));
#26845=DIRECTION('',(0.,-1.,0.));
#26846=DIRECTION('center_axis',(0.,-1.,0.));
#26847=DIRECTION('ref_axis',(0.707106781186546,0.,0.707106781186549));
#26848=DIRECTION('',(0.,-0.382683432365069,0.923879532511295));
#26849=DIRECTION('',(-0.923879532511281,0.382683432365105,-3.20452464650474E-14));
#26850=DIRECTION('center_axis',(0.,-1.,0.));
#26851=DIRECTION('ref_axis',(0.707106781186546,0.,0.707106781186549));
#26852=DIRECTION('center_axis',(0.,0.923879532511288,0.382683432365086));
#26853=DIRECTION('ref_axis',(0.,-0.382683432365086,0.923879532511288));
#26854=DIRECTION('',(0.,-0.382683432365093,0.923879532511285));
#26855=DIRECTION('',(-1.,0.,0.));
#26856=DIRECTION('center_axis',(0.,-1.,0.));
#26857=DIRECTION('ref_axis',(-0.707106781186548,0.,0.707106781186547));
#26858=DIRECTION('',(-0.923879532511289,-0.382683432365085,0.));
#26859=DIRECTION('center_axis',(0.,-1.,0.));
#26860=DIRECTION('ref_axis',(-0.707106781186549,0.,0.707106781186547));
#26861=DIRECTION('center_axis',(-0.382683432365107,0.92387953251128,0.));
#26862=DIRECTION('ref_axis',(0.,0.,1.));
#26863=DIRECTION('',(-0.923879532511281,-0.382683432365103,0.));
#26864=DIRECTION('',(0.,0.,-1.));
#26865=DIRECTION('center_axis',(0.,-1.,0.));
#26866=DIRECTION('ref_axis',(-0.707106781186548,-2.15323663608327E-16,-0.707106781186547));
#26867=DIRECTION('',(0.,-0.382683432365098,-0.923879532511283));
#26868=DIRECTION('center_axis',(0.,1.,-5.80212178386226E-16));
#26869=DIRECTION('ref_axis',(-0.707106781186548,-4.10271965863919E-16,-0.707106781186547));
#26870=DIRECTION('center_axis',(0.,-1.,0.));
#26871=DIRECTION('ref_axis',(-0.707106781186548,0.,-0.707106781186548));
#26872=DIRECTION('center_axis',(0.,0.923879532511284,-0.382683432365097));
#26873=DIRECTION('ref_axis',(0.,0.382683432365097,0.923879532511284));
#26874=DIRECTION('',(0.,-0.382683432365097,-0.923879532511284));
#26875=DIRECTION('',(-1.,0.,0.));
#26876=DIRECTION('',(1.,0.,0.));
#26877=DIRECTION('center_axis',(0.,-1.,0.));
#26878=DIRECTION('ref_axis',(0.707106781186548,0.,-0.707106781186547));
#26879=DIRECTION('',(0.923879532511284,-0.382683432365097,8.01131161626203E-15));
#26880=DIRECTION('center_axis',(-2.90106089193113E-16,1.,-2.90106089193113E-16));
#26881=DIRECTION('ref_axis',(0.707106781186548,0.,-0.707106781186547));
#26882=DIRECTION('center_axis',(0.,-1.,0.));
#26883=DIRECTION('ref_axis',(0.707106781186548,0.,-0.707106781186548));
#26884=DIRECTION('center_axis',(0.382683432365107,0.92387953251128,0.));
#26885=DIRECTION('ref_axis',(0.,0.,1.));
#26886=DIRECTION('',(0.,0.,-1.));
#26887=DIRECTION('',(0.,0.,1.));
#26888=DIRECTION('center_axis',(0.,0.707106781186547,-0.707106781186549));
#26889=DIRECTION('ref_axis',(-1.,0.,0.));
#26890=DIRECTION('',(0.,-0.707106781186548,-0.707106781186548));
#26891=DIRECTION('',(0.,-0.707106781186549,-0.707106781186547));
#26892=DIRECTION('center_axis',(0.,-1.,0.));
#26893=DIRECTION('ref_axis',(0.707106781186548,0.,-0.707106781186548));
#26894=DIRECTION('',(0.707106781186548,-0.707106781186548,0.));
#26895=DIRECTION('center_axis',(0.707106781186549,0.707106781186547,0.));
#26896=DIRECTION('ref_axis',(0.,0.,-1.));
#26897=DIRECTION('center_axis',(0.,1.,0.));
#26898=DIRECTION('ref_axis',(0.,0.,1.));
#26899=DIRECTION('center_axis',(0.,1.,0.));
#26900=DIRECTION('ref_axis',(1.,0.,0.));
#26901=DIRECTION('center_axis',(0.,-1.,0.));
#26902=DIRECTION('ref_axis',(1.,0.,0.));
#26903=DIRECTION('center_axis',(0.,1.,0.));
#26904=DIRECTION('ref_axis',(1.,0.,0.));
#26905=DIRECTION('',(-0.707106781186547,-0.707106781186547,8.65956056235493E-17));
#26906=DIRECTION('center_axis',(0.,-1.,0.));
#26907=DIRECTION('ref_axis',(1.,0.,0.));
#26908=DIRECTION('center_axis',(0.,-1.,0.));
#26909=DIRECTION('ref_axis',(1.,0.,0.));
#26910=DIRECTION('center_axis',(0.,-1.,0.));
#26911=DIRECTION('ref_axis',(1.,0.,0.));
#26912=DIRECTION('',(0.,-1.,0.));
#26913=DIRECTION('center_axis',(0.,1.,0.));
#26914=DIRECTION('ref_axis',(0.,0.,1.));
#26915=DIRECTION('center_axis',(0.,1.,0.));
#26916=DIRECTION('ref_axis',(1.,0.,0.));
#26917=DIRECTION('center_axis',(0.,-1.,0.));
#26918=DIRECTION('ref_axis',(1.,0.,0.));
#26919=DIRECTION('',(-0.923879532511285,0.382683432365093,-1.1314261122877E-16));
#26920=DIRECTION('center_axis',(0.,1.,0.));
#26921=DIRECTION('ref_axis',(1.,0.,0.));
#26922=DIRECTION('',(0.707106781186546,-0.707106781186549,-8.65956056235491E-17));
#26923=DIRECTION('center_axis',(0.,1.,6.68564742231361E-17));
#26924=DIRECTION('ref_axis',(1.,0.,0.));
#26925=DIRECTION('center_axis',(0.,1.,0.));
#26926=DIRECTION('ref_axis',(1.,0.,0.));
#26927=DIRECTION('',(0.382683432365088,-0.923879532511287,-4.68652040532628E-17));
#26928=DIRECTION('center_axis',(0.,-1.,0.));
#26929=DIRECTION('ref_axis',(1.,0.,0.));
#26930=DIRECTION('',(-0.857167300702113,-0.515038074910053,-1.04972719113862E-16));
#26931=DIRECTION('center_axis',(0.,-1.,0.));
#26932=DIRECTION('ref_axis',(1.,0.,0.));
#26933=DIRECTION('center_axis',(0.,-1.,0.));
#26934=DIRECTION('ref_axis',(1.,0.,0.));
#26935=DIRECTION('',(0.,-1.,0.));
#26936=DIRECTION('center_axis',(0.,-1.,0.));
#26937=DIRECTION('ref_axis',(1.,0.,0.));
#26938=DIRECTION('center_axis',(0.,-1.,0.));
#26939=DIRECTION('ref_axis',(1.,0.,0.));
#26940=DIRECTION('',(-0.707106781186547,-0.707106781186548,-8.65956056235493E-17));
#26941=DIRECTION('center_axis',(0.,-1.,0.));
#26942=DIRECTION('ref_axis',(1.,0.,0.));
#26943=DIRECTION('',(-0.857167300702113,-0.515038074910053,-1.04972719113862E-16));
#26944=DIRECTION('center_axis',(0.,-1.,0.));
#26945=DIRECTION('ref_axis',(1.,0.,0.));
#26946=DIRECTION('center_axis',(0.,-1.,0.));
#26947=DIRECTION('ref_axis',(1.,0.,0.));
#26948=DIRECTION('',(0.,-1.,0.));
#26949=DIRECTION('center_axis',(0.,-1.,0.));
#26950=DIRECTION('ref_axis',(1.,0.,0.));
#26951=DIRECTION('center_axis',(0.,-1.,0.));
#26952=DIRECTION('ref_axis',(1.,0.,0.));
#26953=DIRECTION('',(-0.707106781186546,-0.707106781186549,-8.65956056235491E-17));
#26954=DIRECTION('center_axis',(0.,-1.,0.));
#26955=DIRECTION('ref_axis',(1.,0.,0.));
#26956=DIRECTION('',(-0.857167300702113,-0.515038074910053,-1.04972719113862E-16));
#26957=DIRECTION('center_axis',(0.,-1.,0.));
#26958=DIRECTION('ref_axis',(1.,0.,0.));
#26959=DIRECTION('center_axis',(0.,-1.,0.));
#26960=DIRECTION('ref_axis',(1.,0.,0.));
#26961=DIRECTION('',(0.,-1.,0.));
#26962=DIRECTION('center_axis',(0.,-1.,0.));
#26963=DIRECTION('ref_axis',(1.,0.,0.));
#26964=DIRECTION('center_axis',(0.,-1.,0.));
#26965=DIRECTION('ref_axis',(1.,0.,0.));
#26966=DIRECTION('',(-0.707106781186546,-0.707106781186549,-8.65956056235491E-17));
#26967=DIRECTION('center_axis',(0.,-1.,0.));
#26968=DIRECTION('ref_axis',(-0.707106781186548,0.,-0.707106781186548));
#26969=DIRECTION('center_axis',(0.707106781186548,-0.707106781186548,0.));
#26970=DIRECTION('ref_axis',(0.,0.,-1.));
#26971=DIRECTION('',(0.707106781186548,0.707106781186548,0.));
#26972=DIRECTION('center_axis',(0.,1.,0.));
#26973=DIRECTION('ref_axis',(0.707106781186548,0.,-0.707106781186548));
#26974=DIRECTION('center_axis',(-1.,0.,0.));
#26975=DIRECTION('ref_axis',(0.,0.,1.));
#26976=DIRECTION('',(0.,-1.,0.));
#26977=DIRECTION('',(0.,1.,0.));
#26978=DIRECTION('center_axis',(0.,1.,0.));
#26979=DIRECTION('ref_axis',(-0.707106781186548,0.,0.707106781186546));
#26980=DIRECTION('',(0.,1.,0.));
#26981=DIRECTION('center_axis',(0.,0.,1.));
#26982=DIRECTION('ref_axis',(1.,0.,0.));
#26983=DIRECTION('center_axis',(0.,1.,0.));
#26984=DIRECTION('ref_axis',(-0.707106781186547,0.,-0.707106781186547));
#32671=CARTESIAN_POINT('',(0.,0.,0.));
#32672=CARTESIAN_POINT('Origin',(5.4,-3.3893933982822,13.9));
#32673=CARTESIAN_POINT('',(5.89,-3.4,13.9));
#32674=CARTESIAN_POINT('',(5.9412132034356,-3.3787867965644,13.9));
#32675=CARTESIAN_POINT('',(5.89,-3.4,13.9));
#32676=CARTESIAN_POINT('',(5.4,-3.3787867965644,14.4412132034356));
#32677=CARTESIAN_POINT('Origin',(5.4,-3.3787867965644,13.9));
#32678=CARTESIAN_POINT('',(5.4,-3.4,14.39));
#32679=CARTESIAN_POINT('',(5.4,-3.3787867965644,14.4412132034356));
#32680=CARTESIAN_POINT('Origin',(5.4,-3.4,13.9));
#32681=CARTESIAN_POINT('Origin',(5.9156066017178,-3.3893933982822,10.));
#32682=CARTESIAN_POINT('',(5.89,-3.4,3.1));
#32683=CARTESIAN_POINT('',(5.9412132034356,-3.3787867965644,3.1));
#32684=CARTESIAN_POINT('',(5.89,-3.4,3.1));
#32685=CARTESIAN_POINT('',(5.9412132034356,-3.3787867965644,10.));
#32686=CARTESIAN_POINT('',(5.89,-3.4,10.));
#32687=CARTESIAN_POINT('Origin',(5.4,-3.3893933982822,3.1));
#32688=CARTESIAN_POINT('',(5.4,-3.4,2.61));
#32689=CARTESIAN_POINT('',(5.4,-3.3787867965644,2.5587867965644));
#32690=CARTESIAN_POINT('',(5.4,-3.4,2.61));
#32691=CARTESIAN_POINT('Origin',(5.4,-3.3787867965644,3.1));
#32692=CARTESIAN_POINT('Origin',(5.4,-3.4,3.1));
#32693=CARTESIAN_POINT('Origin',(1.5,-3.3893933982822,2.5843933982822));
#32694=CARTESIAN_POINT('',(-5.4,-3.4,2.61));
#32695=CARTESIAN_POINT('',(-5.4,-3.3787867965644,2.5587867965644));
#32696=CARTESIAN_POINT('',(-5.4,-3.4,2.61));
#32697=CARTESIAN_POINT('',(1.5,-3.3787867965644,2.5587867965644));
#32698=CARTESIAN_POINT('',(1.5,-3.4,2.61));
#32699=CARTESIAN_POINT('Origin',(-5.4,-3.3893933982822,3.1));
#32700=CARTESIAN_POINT('',(-5.89,-3.4,3.1));
#32701=CARTESIAN_POINT('',(-5.9412132034356,-3.3787867965644,3.1));
#32702=CARTESIAN_POINT('',(-5.89,-3.4,3.1));
#32703=CARTESIAN_POINT('Origin',(-5.4,-3.3787867965644,3.1));
#32704=CARTESIAN_POINT('Origin',(-5.4,-3.4,3.1));
#32705=CARTESIAN_POINT('Origin',(-5.9156066017178,-3.3893933982822,7.));
#32706=CARTESIAN_POINT('',(-5.89,-3.4,13.9));
#32707=CARTESIAN_POINT('',(-5.9412132034356,-3.3787867965644,13.9));
#32708=CARTESIAN_POINT('',(-5.89,-3.4,13.9));
#32709=CARTESIAN_POINT('',(-5.9412132034356,-3.3787867965644,7.));
#32710=CARTESIAN_POINT('',(-5.89,-3.4,7.));
#32711=CARTESIAN_POINT('Origin',(-5.4,-3.3893933982822,13.9));
#32712=CARTESIAN_POINT('',(-5.4,-3.4,14.39));
#32713=CARTESIAN_POINT('',(-5.4,-3.3787867965644,14.4412132034356));
#32714=CARTESIAN_POINT('',(-5.4,-3.4,14.39));
#32715=CARTESIAN_POINT('Origin',(-5.4,-3.3787867965644,13.9));
#32716=CARTESIAN_POINT('Origin',(-5.4,-3.4,13.9));
#32717=CARTESIAN_POINT('Origin',(-1.5,-3.3893933982822,14.4156066017178));
#32718=CARTESIAN_POINT('',(-1.5,-3.3787867965644,14.4412132034356));
#32719=CARTESIAN_POINT('',(-1.5,-3.4,14.39));
#32720=CARTESIAN_POINT('Origin',(-5.96,-3.36,5.5));
#32721=CARTESIAN_POINT('',(-5.9787867965644,-3.3412132034356,13.9));
#32722=CARTESIAN_POINT('',(-5.92,-3.4,13.9));
#32723=CARTESIAN_POINT('',(-5.9787867965644,-3.3412132034356,3.1));
#32724=CARTESIAN_POINT('',(-5.9787867965644,-3.3412132034356,4.));
#32725=CARTESIAN_POINT('',(-5.92,-3.4,3.1));
#32726=CARTESIAN_POINT('Origin',(-5.4,-3.36,13.9));
#32727=CARTESIAN_POINT('',(-5.4,-3.3412132034356,14.4787867965644));
#32728=CARTESIAN_POINT('',(-5.4,-3.4,14.42));
#32729=CARTESIAN_POINT('Origin',(-5.4,-3.3412132034356,13.9));
#32730=CARTESIAN_POINT('Origin',(-3.,-3.36,14.46));
#32731=CARTESIAN_POINT('',(5.4,-3.3412132034356,14.4787867965644));
#32732=CARTESIAN_POINT('',(5.4,-3.32,14.5));
#32733=CARTESIAN_POINT('',(-4.5,-3.3412132034356,14.4787867965644));
#32734=CARTESIAN_POINT('Origin',(5.4,-3.36,13.9));
#32735=CARTESIAN_POINT('',(5.9787867965644,-3.3412132034356,13.9));
#32736=CARTESIAN_POINT('',(5.92,-3.4,13.9));
#32737=CARTESIAN_POINT('Origin',(5.4,-3.3412132034356,13.9));
#32738=CARTESIAN_POINT('Origin',(0.,-3.4,8.5));
#32739=CARTESIAN_POINT('',(3.805,-3.4,8.5));
#32740=CARTESIAN_POINT('Origin',(0.,-3.4,8.5));
#32741=CARTESIAN_POINT('',(-0.255000000000001,-3.4,3.9));
#32742=CARTESIAN_POINT('Origin',(-8.45006291411674E-16,-3.4,3.9));
#32743=CARTESIAN_POINT('',(-3.50769119345812,-3.4,11.7526911934581));
#32744=CARTESIAN_POINT('Origin',(-3.25269119345812,-3.4,11.7526911934581));
#32745=CARTESIAN_POINT('',(2.99769119345812,-3.4,11.7526911934581));
#32746=CARTESIAN_POINT('Origin',(3.25269119345812,-3.4,11.7526911934581));
#32747=CARTESIAN_POINT('Origin',(4.5,-3.3156066017178,2.5106066017178));
#32748=CARTESIAN_POINT('',(5.4,-3.29,2.5));
#32749=CARTESIAN_POINT('',(5.4,-3.3412132034356,2.5212132034356));
#32750=CARTESIAN_POINT('',(5.4,-3.29,2.5));
#32751=CARTESIAN_POINT('',(-5.4,-3.3412132034356,2.5212132034356));
#32752=CARTESIAN_POINT('',(4.5,-3.3412132034356,2.5212132034356));
#32753=CARTESIAN_POINT('',(-5.4,-3.29,2.5));
#32754=CARTESIAN_POINT('',(-5.4,-3.3412132034356,2.5212132034356));
#32755=CARTESIAN_POINT('',(4.5,-3.29,2.5));
#32756=CARTESIAN_POINT('Origin',(5.4,-3.3156066017178,3.1));
#32757=CARTESIAN_POINT('',(6.,-3.29,3.1));
#32758=CARTESIAN_POINT('',(5.9787867965644,-3.3412132034356,3.1));
#32759=CARTESIAN_POINT('',(6.,-3.29,3.1));
#32760=CARTESIAN_POINT('Origin',(5.4,-3.3412132034356,3.1));
#32761=CARTESIAN_POINT('Origin',(5.4,-3.29,3.1));
#32762=CARTESIAN_POINT('Origin',(5.9893933982822,-3.3156066017178,13.));
#32763=CARTESIAN_POINT('',(6.,-3.29,13.9));
#32764=CARTESIAN_POINT('',(6.,-3.29,13.9));
#32765=CARTESIAN_POINT('',(5.9787867965644,-3.3412132034356,13.));
#32766=CARTESIAN_POINT('',(6.,-3.29,13.));
#32767=CARTESIAN_POINT('Origin',(5.4,-3.3156066017178,13.9));
#32768=CARTESIAN_POINT('',(5.4,-3.29,14.5));
#32769=CARTESIAN_POINT('',(5.4,-3.29,14.5));
#32770=CARTESIAN_POINT('Origin',(5.4,-3.29,13.9));
#32771=CARTESIAN_POINT('Origin',(-4.5,-3.3156066017178,14.4893933982822));
#32772=CARTESIAN_POINT('',(-5.4,-3.29,14.5));
#32773=CARTESIAN_POINT('',(-5.4,-3.29,14.5));
#32774=CARTESIAN_POINT('',(-4.5,-3.29,14.5));
#32775=CARTESIAN_POINT('Origin',(-5.4,-3.3156066017178,13.9));
#32776=CARTESIAN_POINT('',(-6.,-3.29,13.9));
#32777=CARTESIAN_POINT('',(-6.,-3.29,13.9));
#32778=CARTESIAN_POINT('Origin',(-5.4,-3.29,13.9));
#32779=CARTESIAN_POINT('Origin',(-5.9893933982822,-3.3156066017178,4.));
#32780=CARTESIAN_POINT('',(-6.,-3.29,3.1));
#32781=CARTESIAN_POINT('',(-6.,-3.29,3.1));
#32782=CARTESIAN_POINT('',(-6.,-3.29,4.));
#32783=CARTESIAN_POINT('Origin',(-5.4,-3.3156066017178,3.1));
#32784=CARTESIAN_POINT('Origin',(-5.4,-3.3412132034356,3.1));
#32785=CARTESIAN_POINT('Origin',(-5.4,-3.29,3.1));
#32786=CARTESIAN_POINT('Origin',(5.4,-3.4,13.9));
#32787=CARTESIAN_POINT('',(6.,-1.71,13.9));
#32788=CARTESIAN_POINT('',(6.,-3.4,13.9));
#32789=CARTESIAN_POINT('',(5.4,-1.71,14.5));
#32790=CARTESIAN_POINT('Origin',(5.4,-1.71,13.9));
#32791=CARTESIAN_POINT('',(5.4,-3.4,14.5));
#32792=CARTESIAN_POINT('Origin',(6.,-3.4,14.5));
#32793=CARTESIAN_POINT('',(6.,-1.71,3.1));
#32794=CARTESIAN_POINT('',(6.,-3.4,3.1));
#32795=CARTESIAN_POINT('',(6.,-1.71,13.));
#32796=CARTESIAN_POINT('Origin',(5.4,-3.4,3.1));
#32797=CARTESIAN_POINT('',(5.4,-1.71,2.5));
#32798=CARTESIAN_POINT('',(5.4,-3.4,2.5));
#32799=CARTESIAN_POINT('Origin',(5.4,-1.71,3.1));
#32800=CARTESIAN_POINT('Origin',(6.,-3.4,2.5));
#32801=CARTESIAN_POINT('',(-5.4,-1.71,2.5));
#32802=CARTESIAN_POINT('',(-5.4,-3.4,2.5));
#32803=CARTESIAN_POINT('',(4.5,-1.71,2.5));
#32804=CARTESIAN_POINT('Origin',(-5.4,-3.36,3.1));
#32805=CARTESIAN_POINT('',(-5.4,-3.4,2.58));
#32806=CARTESIAN_POINT('Origin',(3.,-3.36,2.54));
#32807=CARTESIAN_POINT('',(5.4,-3.4,2.58));
#32808=CARTESIAN_POINT('Origin',(5.4,-1.6843933982822,13.9));
#32809=CARTESIAN_POINT('',(5.9787867965644,-1.6587867965644,13.9));
#32810=CARTESIAN_POINT('',(6.,-1.71,13.9));
#32811=CARTESIAN_POINT('',(5.4,-1.6587867965644,14.4787867965644));
#32812=CARTESIAN_POINT('Origin',(5.4,-1.6587867965644,13.9));
#32813=CARTESIAN_POINT('',(5.4,-1.6587867965644,14.4787867965644));
#32814=CARTESIAN_POINT('Origin',(5.9893933982822,-1.6843933982822,13.));
#32815=CARTESIAN_POINT('',(5.9787867965644,-1.6587867965644,3.1));
#32816=CARTESIAN_POINT('',(6.,-1.71,3.1));
#32817=CARTESIAN_POINT('',(5.9787867965644,-1.6587867965644,13.));
#32818=CARTESIAN_POINT('Origin',(5.4,-1.6843933982822,3.1));
#32819=CARTESIAN_POINT('',(5.4,-1.6587867965644,2.5212132034356));
#32820=CARTESIAN_POINT('',(5.4,-1.71,2.5));
#32821=CARTESIAN_POINT('Origin',(5.4,-1.6587867965644,3.1));
#32822=CARTESIAN_POINT('Origin',(4.5,-1.6843933982822,2.5106066017178));
#32823=CARTESIAN_POINT('',(-5.4,-1.6587867965644,2.5212132034356));
#32824=CARTESIAN_POINT('',(-5.4,-1.71,2.5));
#32825=CARTESIAN_POINT('',(4.5,-1.6587867965644,2.5212132034356));
#32826=CARTESIAN_POINT('Origin',(-5.4,-1.6843933982822,3.1));
#32827=CARTESIAN_POINT('',(-6.,-1.71,3.1));
#32828=CARTESIAN_POINT('',(-5.9787867965644,-1.6587867965644,3.1));
#32829=CARTESIAN_POINT('',(-6.,-1.71,3.1));
#32830=CARTESIAN_POINT('Origin',(-5.4,-1.6587867965644,3.1));
#32831=CARTESIAN_POINT('Origin',(-5.4,-1.71,3.1));
#32832=CARTESIAN_POINT('Origin',(-5.9893933982822,-1.6843933982822,4.));
#32833=CARTESIAN_POINT('',(-6.,-1.71,13.9));
#32834=CARTESIAN_POINT('',(-5.9787867965644,-1.6587867965644,13.9));
#32835=CARTESIAN_POINT('',(-6.,-1.71,13.9));
#32836=CARTESIAN_POINT('',(-5.9787867965644,-1.6587867965644,4.));
#32837=CARTESIAN_POINT('',(-6.,-1.71,4.));
#32838=CARTESIAN_POINT('Origin',(-5.4,-1.6843933982822,13.9));
#32839=CARTESIAN_POINT('',(-5.4,-1.71,14.5));
#32840=CARTESIAN_POINT('',(-5.4,-1.65878679656441,14.4787867965644));
#32841=CARTESIAN_POINT('',(-5.4,-1.71,14.5));
#32842=CARTESIAN_POINT('Origin',(-5.4,-1.6587867965644,13.9));
#32843=CARTESIAN_POINT('Origin',(-5.4,-1.71,13.9));
#32844=CARTESIAN_POINT('Origin',(-4.5,-1.6843933982822,14.4893933982822));
#32845=CARTESIAN_POINT('',(-4.5,-1.6587867965644,14.4787867965644));
#32846=CARTESIAN_POINT('',(-4.5,-1.71,14.5));
#32847=CARTESIAN_POINT('Origin',(-5.96,-1.64,5.5));
#32848=CARTESIAN_POINT('',(-5.9412132034356,-1.6212132034356,13.9));
#32849=CARTESIAN_POINT('',(-5.92,-1.6,13.9));
#32850=CARTESIAN_POINT('',(-5.9412132034356,-1.6212132034356,3.1));
#32851=CARTESIAN_POINT('',(-5.9412132034356,-1.6212132034356,7.));
#32852=CARTESIAN_POINT('',(-5.92,-1.6,3.1));
#32853=CARTESIAN_POINT('Origin',(-5.4,-1.64,13.9));
#32854=CARTESIAN_POINT('',(-5.4,-1.6212132034356,14.4412132034356));
#32855=CARTESIAN_POINT('',(-5.4,-1.6,14.42));
#32856=CARTESIAN_POINT('Origin',(-5.4,-1.6212132034356,13.9));
#32857=CARTESIAN_POINT('Origin',(-3.,-1.64,14.46));
#32858=CARTESIAN_POINT('',(5.4,-1.62121320343559,14.4412132034356));
#32859=CARTESIAN_POINT('',(5.4,-1.6,14.42));
#32860=CARTESIAN_POINT('',(-1.5,-1.6212132034356,14.4412132034356));
#32861=CARTESIAN_POINT('Origin',(5.4,-1.64,13.9));
#32862=CARTESIAN_POINT('',(5.9412132034356,-1.6212132034356,13.9));
#32863=CARTESIAN_POINT('',(6.,-1.68,13.9));
#32864=CARTESIAN_POINT('Origin',(5.4,-1.6212132034356,13.9));
#32865=CARTESIAN_POINT('Origin',(0.,-3.385,8.5));
#32866=CARTESIAN_POINT('',(3.775,-3.37,8.5));
#32867=CARTESIAN_POINT('',(3.79,-3.385,8.5));
#32868=CARTESIAN_POINT('',(-3.775,-3.37,8.5));
#32869=CARTESIAN_POINT('Origin',(0.,-3.37,8.5));
#32870=CARTESIAN_POINT('Origin',(0.,-3.37,8.5));
#32871=CARTESIAN_POINT('Origin',(0.,-2.8,8.5));
#32872=CARTESIAN_POINT('',(-3.775,-2.2,8.5));
#32873=CARTESIAN_POINT('Origin',(0.,-2.2,8.5));
#32874=CARTESIAN_POINT('',(-3.775,-2.8,8.5));
#32875=CARTESIAN_POINT('Origin',(5.4,-1.6106066017178,13.9));
#32876=CARTESIAN_POINT('',(5.4,-1.6,14.39));
#32877=CARTESIAN_POINT('',(5.4,-1.6,14.39));
#32878=CARTESIAN_POINT('',(5.89,-1.6,13.9));
#32879=CARTESIAN_POINT('',(5.9412132034356,-1.6212132034356,13.9));
#32880=CARTESIAN_POINT('Origin',(5.4,-1.6,13.9));
#32881=CARTESIAN_POINT('Origin',(-1.5,-1.6106066017178,14.4156066017178));
#32882=CARTESIAN_POINT('',(-5.4,-1.6,14.39));
#32883=CARTESIAN_POINT('',(-5.4,-1.6,14.39));
#32884=CARTESIAN_POINT('',(-1.5,-1.6,14.39));
#32885=CARTESIAN_POINT('Origin',(-5.4,-1.6106066017178,13.9));
#32886=CARTESIAN_POINT('',(-5.89,-1.6,13.9));
#32887=CARTESIAN_POINT('',(-5.89,-1.6,13.9));
#32888=CARTESIAN_POINT('Origin',(-5.4,-1.6,13.9));
#32889=CARTESIAN_POINT('Origin',(-5.9156066017178,-1.6106066017178,7.));
#32890=CARTESIAN_POINT('',(-5.89,-1.6,3.1));
#32891=CARTESIAN_POINT('',(-5.89,-1.6,3.1));
#32892=CARTESIAN_POINT('',(-5.89,-1.6,7.));
#32893=CARTESIAN_POINT('Origin',(-5.4,-1.6106066017178,3.1));
#32894=CARTESIAN_POINT('',(-5.4,-1.6,2.61));
#32895=CARTESIAN_POINT('',(-5.4,-1.6212132034356,2.5587867965644));
#32896=CARTESIAN_POINT('',(-5.4,-1.6,2.61));
#32897=CARTESIAN_POINT('Origin',(-5.4,-1.6212132034356,3.1));
#32898=CARTESIAN_POINT('Origin',(-5.4,-1.6,3.1));
#32899=CARTESIAN_POINT('Origin',(1.5,-1.6106066017178,2.5843933982822));
#32900=CARTESIAN_POINT('',(5.4,-1.6,2.61));
#32901=CARTESIAN_POINT('',(5.4,-1.6212132034356,2.5587867965644));
#32902=CARTESIAN_POINT('',(5.4,-1.6,2.61));
#32903=CARTESIAN_POINT('',(1.5,-1.6212132034356,2.5587867965644));
#32904=CARTESIAN_POINT('',(1.5,-1.6,2.61));
#32905=CARTESIAN_POINT('Origin',(5.4,-1.6106066017178,3.1));
#32906=CARTESIAN_POINT('',(5.89,-1.6,3.1));
#32907=CARTESIAN_POINT('',(5.9412132034356,-1.6212132034356,3.1));
#32908=CARTESIAN_POINT('',(5.89,-1.6,3.1));
#32909=CARTESIAN_POINT('Origin',(5.4,-1.6212132034356,3.1));
#32910=CARTESIAN_POINT('Origin',(5.4,-1.6,3.1));
#32911=CARTESIAN_POINT('Origin',(5.9156066017178,-1.6106066017178,10.));
#32912=CARTESIAN_POINT('',(5.9412132034356,-1.6212132034356,10.));
#32913=CARTESIAN_POINT('',(5.89,-1.6,10.));
#32914=CARTESIAN_POINT('Origin',(3.,-1.64,2.54));
#32915=CARTESIAN_POINT('',(-5.4,-1.6,2.58));
#32916=CARTESIAN_POINT('',(5.4,-1.6,2.58));
#32917=CARTESIAN_POINT('Origin',(5.4,-1.64,3.1));
#32918=CARTESIAN_POINT('',(5.92,-1.6,3.1));
#32919=CARTESIAN_POINT('Origin',(5.96,-1.64,11.5));
#32920=CARTESIAN_POINT('Origin',(0.,-1.6,8.5));
#32921=CARTESIAN_POINT('',(-3.38,-1.6,8.5));
#32922=CARTESIAN_POINT('Origin',(0.,-1.6,8.5));
#32923=CARTESIAN_POINT('Origin',(0.,-2.185,8.5));
#32924=CARTESIAN_POINT('',(-3.3,-2.17,8.5));
#32925=CARTESIAN_POINT('Origin',(0.,-2.17,8.5));
#32926=CARTESIAN_POINT('',(-3.33,-2.2,8.5));
#32927=CARTESIAN_POINT('',(-3.315,-2.185,8.5));
#32928=CARTESIAN_POINT('Origin',(0.,-2.2,8.5));
#32929=CARTESIAN_POINT('Origin',(0.,-2.5,8.5));
#32930=CARTESIAN_POINT('',(-3.3,-1.68,8.5));
#32931=CARTESIAN_POINT('Origin',(0.,-1.68,8.5));
#32932=CARTESIAN_POINT('',(-3.3,-2.5,8.5));
#32933=CARTESIAN_POINT('Origin',(3.775,-2.2,8.5));
#32934=CARTESIAN_POINT('Origin',(0.,-1.6106066017178,8.5));
#32935=CARTESIAN_POINT('',(-3.3287867965644,-1.6212132034356,8.5));
#32936=CARTESIAN_POINT('Origin',(0.,-1.6212132034356,8.5));
#32937=CARTESIAN_POINT('',(-3.3543933982822,-1.6106066017178,8.5));
#32938=CARTESIAN_POINT('Origin',(0.,-1.625,8.5));
#32939=CARTESIAN_POINT('',(-3.3212132034356,-1.6287867965644,8.5));
#32940=CARTESIAN_POINT('',(-3.325,-1.625,8.5));
#32941=CARTESIAN_POINT('Origin',(0.,-1.6287867965644,8.5));
#32942=CARTESIAN_POINT('Origin',(0.,-1.6543933982822,8.5));
#32943=CARTESIAN_POINT('',(-3.3106066017178,-1.6543933982822,8.5));
#32944=CARTESIAN_POINT('Origin',(-8.45006291411674E-16,-2.33841178654967,
3.9));
#32945=CARTESIAN_POINT('',(-8.45006291411674E-16,-2.27682357309935,3.9));
#32946=CARTESIAN_POINT('',(-0.205000000000001,-2.4,3.9));
#32947=CARTESIAN_POINT('',(-0.102500000000001,-2.33841178654967,3.9));
#32948=CARTESIAN_POINT('Origin',(-8.45006291411674E-16,-2.4,3.9));
#32949=CARTESIAN_POINT('Origin',(-8.45006291411674E-16,-2.875,3.9));
#32950=CARTESIAN_POINT('',(-0.205000000000001,-3.35,3.9));
#32951=CARTESIAN_POINT('',(-0.205000000000001,-2.875,3.9));
#32952=CARTESIAN_POINT('Origin',(-8.45006291411674E-16,-3.35,3.9));
#32953=CARTESIAN_POINT('Origin',(-8.45006291411674E-16,-3.4,3.9));
#32954=CARTESIAN_POINT('',(-0.255000000000001,-3.4,3.9));
#32955=CARTESIAN_POINT('Origin',(-3.25269119345812,-2.33841178654967,11.7526911934581));
#32956=CARTESIAN_POINT('',(-3.25269119345812,-2.27682357309935,11.7526911934581));
#32957=CARTESIAN_POINT('',(-3.45769119345812,-2.4,11.7526911934581));
#32958=CARTESIAN_POINT('',(-3.35519119345812,-2.33841178654967,11.7526911934581));
#32959=CARTESIAN_POINT('Origin',(-3.25269119345812,-2.4,11.7526911934581));
#32960=CARTESIAN_POINT('Origin',(-3.25269119345812,-2.875,11.7526911934581));
#32961=CARTESIAN_POINT('',(-3.45769119345812,-3.35,11.7526911934581));
#32962=CARTESIAN_POINT('',(-3.45769119345812,-2.875,11.7526911934581));
#32963=CARTESIAN_POINT('Origin',(-3.25269119345812,-3.35,11.7526911934581));
#32964=CARTESIAN_POINT('Origin',(-3.25269119345812,-3.4,11.7526911934581));
#32965=CARTESIAN_POINT('',(-3.50769119345812,-3.4,11.7526911934581));
#32966=CARTESIAN_POINT('Origin',(3.25269119345812,-2.33841178654967,11.7526911934581));
#32967=CARTESIAN_POINT('',(3.25269119345812,-2.27682357309935,11.7526911934581));
#32968=CARTESIAN_POINT('',(3.04769119345812,-2.4,11.7526911934581));
#32969=CARTESIAN_POINT('',(3.15019119345812,-2.33841178654967,11.7526911934581));
#32970=CARTESIAN_POINT('Origin',(3.25269119345812,-2.4,11.7526911934581));
#32971=CARTESIAN_POINT('Origin',(3.25269119345812,-2.875,11.7526911934581));
#32972=CARTESIAN_POINT('',(3.04769119345812,-3.35,11.7526911934581));
#32973=CARTESIAN_POINT('',(3.04769119345812,-2.875,11.7526911934581));
#32974=CARTESIAN_POINT('Origin',(3.25269119345812,-3.35,11.7526911934581));
#32975=CARTESIAN_POINT('Origin',(3.25269119345812,-3.4,11.7526911934581));
#32976=CARTESIAN_POINT('',(2.99769119345812,-3.4,11.7526911934581));
#32977=CARTESIAN_POINT('Origin',(-5.4,-1.64,3.1));
#32978=CARTESIAN_POINT('Origin',(5.96,-3.36,11.5));
#32979=CARTESIAN_POINT('',(5.92,-3.4,3.1));
#32980=CARTESIAN_POINT('Origin',(5.4,-3.36,3.1));
#32981=CARTESIAN_POINT('Origin',(-6.,-3.4,2.5));
#32982=CARTESIAN_POINT('',(-6.,-3.4,13.9));
#32983=CARTESIAN_POINT('',(-6.,-3.4,3.1));
#32984=CARTESIAN_POINT('Origin',(-5.4,-3.4,13.9));
#32985=CARTESIAN_POINT('',(-5.4,-3.4,14.5));
#32986=CARTESIAN_POINT('Origin',(-6.,-3.4,14.5));
#32987=CARTESIAN_POINT('Origin',(-5.4,-3.4,3.1));
#53618=UNCERTAINTY_MEASURE_WITH_UNIT(LENGTH_MEASURE(0.001),#53651,
'DISTANCE_ACCURACY_VALUE',
'Maximum model space distance between geometric entities at asserted c
onnectivities');
#53632=UNCERTAINTY_MEASURE_WITH_UNIT(LENGTH_MEASURE(0.001),#53651,
'DISTANCE_ACCURACY_VALUE',
'Maximum model space distance between geometric entities at asserted c
onnectivities');
#53636=(
GEOMETRIC_REPRESENTATION_CONTEXT(3)
GLOBAL_UNCERTAINTY_ASSIGNED_CONTEXT((#53618))
GLOBAL_UNIT_ASSIGNED_CONTEXT((#53651,#53653,#53654))
REPRESENTATION_CONTEXT('','3D')
);
#53650=(
GEOMETRIC_REPRESENTATION_CONTEXT(3)
GLOBAL_UNCERTAINTY_ASSIGNED_CONTEXT((#53632))
GLOBAL_UNIT_ASSIGNED_CONTEXT((#53651,#53653,#53654))
REPRESENTATION_CONTEXT('','3D')
);
#53651=(
LENGTH_UNIT()
NAMED_UNIT(*)
SI_UNIT(.CENTI.,.METRE.)
);
#53653=(
NAMED_UNIT(*)
PLANE_ANGLE_UNIT()
SI_UNIT($,.RADIAN.)
);
#53654=(
NAMED_UNIT(*)
SI_UNIT($,.STERADIAN.)
SOLID_ANGLE_UNIT()
);
#53658=SHAPE_DEFINITION_REPRESENTATION(#53675,#53726);
#53675=PRODUCT_DEFINITION_SHAPE('',$,#53744);
#53726=SHAPE_REPRESENTATION('',(#23856),#53636);
#53740=PRODUCT_DEFINITION_CONTEXT('part definition',#53793,'design');
#53744=PRODUCT_DEFINITION('2026-10-18-22-44-34-542',
'03_Front_Kinematic_Cell_Alignment_Frame',#53761,#53740);
#53761=PRODUCT_DEFINITION_FORMATION('',$,#53798);
#53793=APPLICATION_CONTEXT(
'Core Data for Automotive Mechanical Design Process');
#53794=PRODUCT_CONTEXT('part definition',#53793,'mechanical');
#53798=PRODUCT('2026-10-18-22-44-34-542',
'03_Front_Kinematic_Cell_Alignment_Frame',$,(#53794));
#53931=COLOUR_RGB('Dark Blue',0.08,0.2,0.34);
#53932=FILL_AREA_STYLE_COLOUR('',#53931);
#53933=FILL_AREA_STYLE('',(#53932));
#53934=SURFACE_STYLE_FILL_AREA(#53933);
#53935=SURFACE_SIDE_STYLE('',(#53934));
#53936=SURFACE_STYLE_USAGE(.BOTH.,#53935);
#53937=PRESENTATION_STYLE_ASSIGNMENT((#53936));
ENDSEC;
END-ISO-10303-21;
